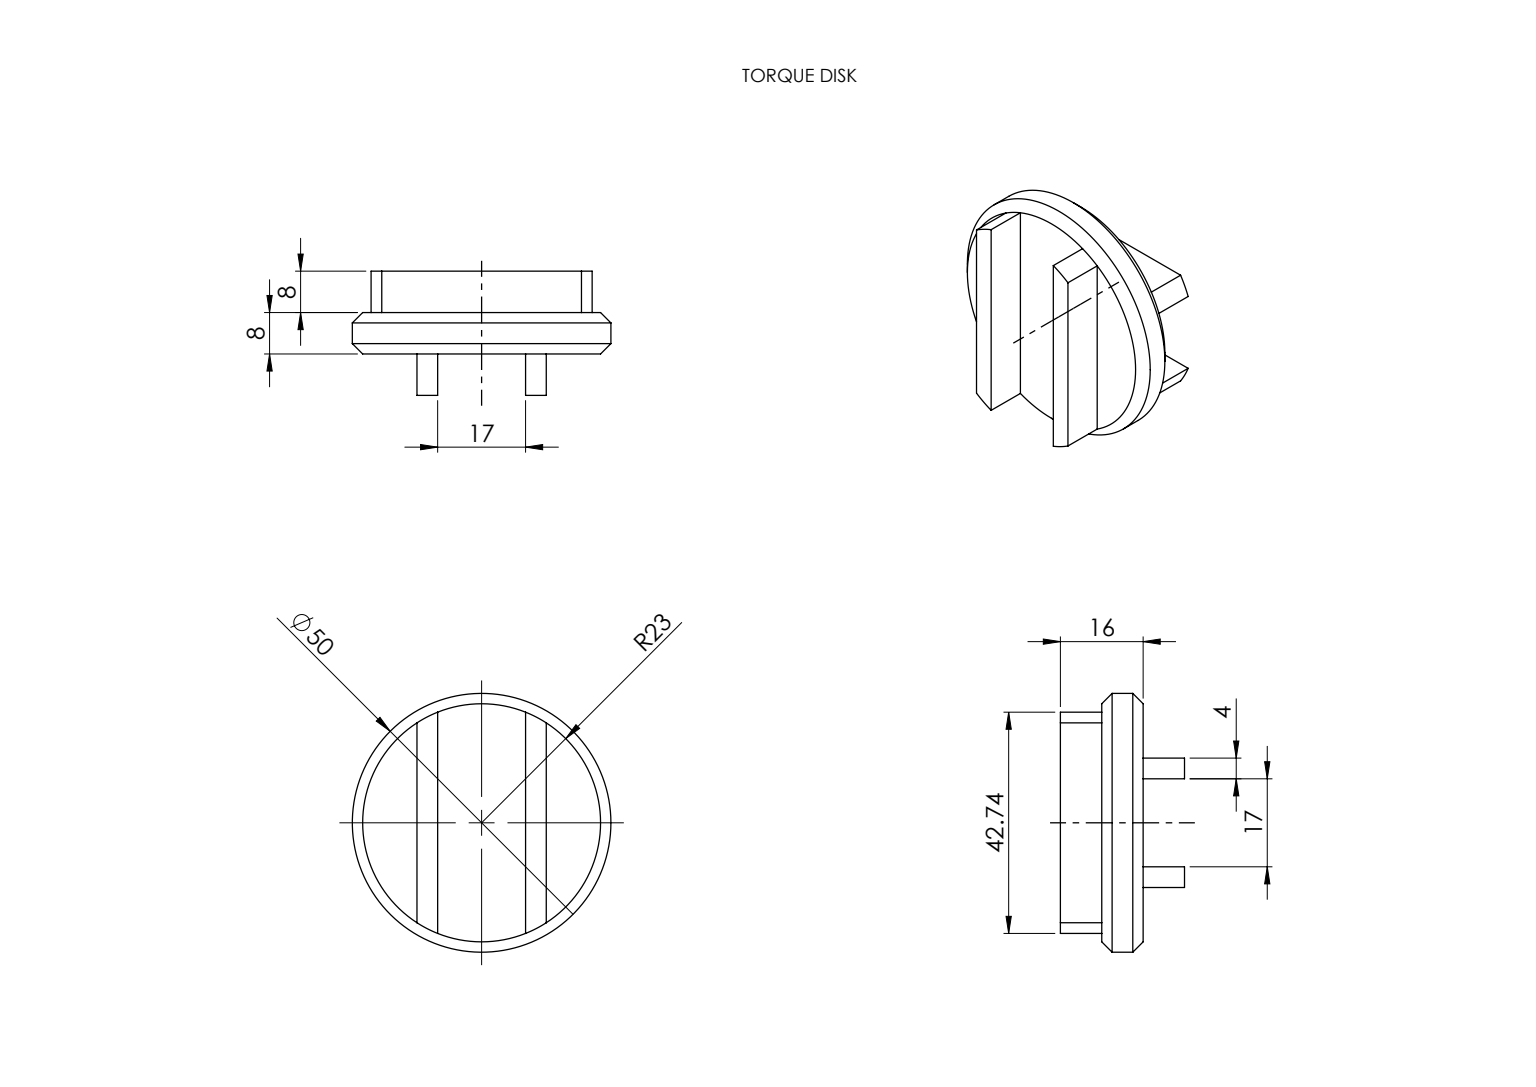
ISO-10303-21;
HEADER;
FILE_DESCRIPTION (('STEP AP214'),
    '1' );
FILE_NAME ('torque disk.step',
    '2026-10-08T14:09:18',
    ( '' ),
    ( '' ),
    'SwSTEP 2.0',
    'SolidWorks 2026',
    '' );
FILE_SCHEMA (( 'AUTOMOTIVE_DESIGN' ));
ENDSEC;

DATA;
#10=( NAMED_UNIT ( * ) PLANE_ANGLE_UNIT ( ) SI_UNIT ( $, .RADIAN. ) );
#11=EDGE_CURVE ( 'NONE', #1059, #406, #4156, .T. ) ;
#17=AXIS2_PLACEMENT_3D ( 'NONE', #2780, #4294, #3843 ) ;
#18=ADVANCED_FACE ( 'NONE', ( #4455 ), #1426, .T. ) ;
#30=ORIENTED_EDGE ( 'NONE', *, *, #808, .T. ) ;
#35=CIRCLE ( 'NONE', #4595, 22.99999999999998934 ) ;
#38=ADVANCED_BREP_SHAPE_REPRESENTATION ( '', ( #2058, #1918 ), #1039 ) ;
#53=EDGE_CURVE ( 'NONE', #754, #3692, #3957, .T. ) ;
#55=ORIENTED_EDGE ( 'NONE', *, *, #2270, .T. ) ;
#61=( NAMED_UNIT ( * ) PLANE_ANGLE_UNIT ( ) SI_UNIT ( $, .RADIAN. ) );
#62=CARTESIAN_POINT ( 'NONE',  ( 0.000000000000000000, 0.000000000000000000, 4.000000000000000000 ) ) ;
#68=EDGE_LOOP ( 'NONE', ( #4400, #3556, #1967, #1620 ) ) ;
#75=ORIENTED_EDGE ( 'NONE', *, *, #4606, .T. ) ;
#76=AXIS2_PLACEMENT_3D ( 'NONE', #1953, #1896, #4546 ) ;
#77=EDGE_LOOP ( 'NONE', ( #2842, #2826, #4730, #3841 ) ) ;
#78=EDGE_CURVE ( 'NONE', #3692, #754, #3167, .T. ) ;
#86=DIRECTION ( 'NONE',  ( 1.000000000000000000, 0.000000000000000000, -0.000000000000000000 ) ) ;
#93=LINE ( 'NONE', #2056, #2959 ) ;
#96=VECTOR ( 'NONE', #306, 1000.000000000000000 ) ;
#119=DIRECTION ( 'NONE',  ( 1.000000000000000000, 0.000000000000000000, 0.000000000000000000 ) ) ;
#123=DIRECTION ( 'NONE',  ( -0.000000000000000000, -0.000000000000000000, -1.000000000000000000 ) ) ;
#125=EDGE_LOOP ( 'NONE', ( #685, #558, #2484, #4035, #4209, #3718, #4513, #747 ) ) ;
#134=DIRECTION ( 'NONE',  ( 0.7071067811865487940, 0.000000000000000000, 0.7071067811865463515 ) ) ;
#152=ORIENTED_EDGE ( 'NONE', *, *, #1724, .T. ) ;
#167=CARTESIAN_POINT ( 'NONE',  ( -12.50000000000000178, 19.30673457630782863, 4.000000000000000000 ) ) ;
#169=AXIS2_PLACEMENT_3D ( 'NONE', #62, #3894, #4293 ) ;
#179=CARTESIAN_POINT ( 'NONE',  ( 23.00000000000000711, 2.939152317953648289E-15, 4.000000000000000000 ) ) ;
#186=DIRECTION ( 'NONE',  ( 1.000000000000000000, -1.106769389831504189E-16, 0.000000000000000000 ) ) ;
#192=ORIENTED_EDGE ( 'NONE', *, *, #1976, .T. ) ;
#200=DIRECTION ( 'NONE',  ( 1.000000000000000000, 0.000000000000000000, 0.000000000000000000 ) ) ;
#203=CARTESIAN_POINT ( 'NONE',  ( 2.853620410115562697E-14, 8.500000000000001776, -12.00000000000000000 ) ) ;
#205=CARTESIAN_POINT ( 'NONE',  ( 0.000000000000000000, 0.000000000000000000, -12.00000000000000000 ) ) ;
#212=VERTEX_POINT ( 'NONE', #756 ) ;
#215=DIRECTION ( 'NONE',  ( -0.000000000000000000, 0.000000000000000000, 1.000000000000000000 ) ) ;
#224=DIRECTION ( 'NONE',  ( -0.000000000000000000, -0.000000000000000000, 1.000000000000000000 ) ) ;
#234=EDGE_CURVE ( 'NONE', #1400, #1443, #448, .T. ) ;
#235=EDGE_LOOP ( 'NONE', ( #4089, #4144 ) ) ;
#246=ORIENTED_EDGE ( 'NONE', *, *, #3864, .T. ) ;
#257=AXIS2_PLACEMENT_3D ( 'NONE', #3512, #3491, #493 ) ;
#272=EDGE_CURVE ( 'NONE', #4859, #4459, #35, .T. ) ;
#283=ORIENTED_EDGE ( 'NONE', *, *, #1551, .T. ) ;
#287=ORIENTED_EDGE ( 'NONE', *, *, #3972, .T. ) ;
#291=DIRECTION ( 'NONE',  ( -1.106769389831504682E-16, -1.000000000000000000, 0.000000000000000000 ) ) ;
#293=FACE_OUTER_BOUND ( 'NONE', #4691, .T. ) ;
#301=CARTESIAN_POINT ( 'NONE',  ( 0.000000000000000000, 0.000000000000000000, 12.00000000000000000 ) ) ;
#302=CARTESIAN_POINT ( 'NONE',  ( 0.000000000000000000, 0.000000000000000000, -12.00000000000000000 ) ) ;
#306=DIRECTION ( 'NONE',  ( 1.000000000000000000, -3.578554360455197734E-15, 0.000000000000000000 ) ) ;
#308=ORIENTED_EDGE ( 'NONE', *, *, #4604, .F. ) ;
#320=PLANE ( 'NONE',  #4355 ) ;
#328=DIRECTION ( 'NONE',  ( -0.000000000000000000, -0.000000000000000000, 1.000000000000000000 ) ) ;
#333=DIRECTION ( 'NONE',  ( 0.000000000000000000, 0.000000000000000000, 1.000000000000000000 ) ) ;
#337=VECTOR ( 'NONE', #2303, 999.9999999999998863 ) ;
#352=ADVANCED_FACE ( 'NONE', ( #4835 ), #4072, .F. ) ;
#372=DIRECTION ( 'NONE',  ( 0.000000000000000000, 0.000000000000000000, 1.000000000000000000 ) ) ;
#374=VERTEX_POINT ( 'NONE', #1802 ) ;
#379=EDGE_CURVE ( 'NONE', #803, #3915, #997, .T. ) ;
#384=DIRECTION ( 'NONE',  ( 1.000000000000000000, -3.578554360455197734E-15, 0.000000000000000000 ) ) ;
#403=CYLINDRICAL_SURFACE ( 'NONE', #418, 23.00000000000000711 ) ;
#406=VERTEX_POINT ( 'NONE', #2208 ) ;
#412=CARTESIAN_POINT ( 'NONE',  ( 0.000000000000000000, 0.000000000000000000, -1.999999999999994893 ) ) ;
#417=FILL_AREA_STYLE ('',( #3127 ) ) ;
#418=AXIS2_PLACEMENT_3D ( 'NONE', #1930, #2739, #4659 ) ;
#421=ADVANCED_FACE ( 'NONE', ( #3011 ), #320, .F. ) ;
#422=DIRECTION ( 'NONE',  ( -0.000000000000000000, -0.000000000000000000, 1.000000000000000000 ) ) ;
#430=EDGE_CURVE ( 'NONE', #3154, #4346, #3398, .T. ) ;
#439=DIRECTION ( 'NONE',  ( -0.000000000000000000, -0.000000000000000000, 1.000000000000000000 ) ) ;
#440=DIRECTION ( 'NONE',  ( 0.000000000000000000, 0.000000000000000000, 1.000000000000000000 ) ) ;
#442=EDGE_LOOP ( 'NONE', ( #1911, #3869, #3953, #75 ) ) ;
#444=DIRECTION ( 'NONE',  ( -0.000000000000000000, -0.000000000000000000, -1.000000000000000000 ) ) ;
#445=CARTESIAN_POINT ( 'NONE',  ( 0.000000000000000000, 0.000000000000000000, -12.00000000000000000 ) ) ;
#448=CIRCLE ( 'NONE', #1077, 22.99999999999998934 ) ;
#450=EDGE_CURVE ( 'NONE', #1059, #4052, #4677, .T. ) ;
#451=VERTEX_POINT ( 'NONE', #717 ) ;
#453=CARTESIAN_POINT ( 'NONE',  ( 0.000000000000000000, 0.000000000000000000, 4.000000000000000000 ) ) ;
#454=DIRECTION ( 'NONE',  ( -0.000000000000000000, 0.000000000000000000, 1.000000000000000000 ) ) ;
#456=ORIENTED_EDGE ( 'NONE', *, *, #4832, .F. ) ;
#458=LINE ( 'NONE', #766, #3279 ) ;
#470=CARTESIAN_POINT ( 'NONE',  ( 12.50000000000000178, 19.30673457630782863, 12.00000000000000000 ) ) ;
#471=FACE_OUTER_BOUND ( 'NONE', #854, .T. ) ;
#490=LINE ( 'NONE', #2006, #2180 ) ;
#493=DIRECTION ( 'NONE',  ( 1.000000000000000000, 0.000000000000000000, -0.000000000000000000 ) ) ;
#499=ORIENTED_EDGE ( 'NONE', *, *, #2997, .T. ) ;
#501=CARTESIAN_POINT ( 'NONE',  ( -12.49999999999999822, -19.30673457630782863, 12.00000000000000000 ) ) ;
#505=AXIS2_PLACEMENT_3D ( 'NONE', #2463, #2918, #1335 ) ;
#514=CARTESIAN_POINT ( 'NONE',  ( 8.500000000000003553, 21.37171027316251681, 12.00000000000000000 ) ) ;
#533=ORIENTED_EDGE ( 'NONE', *, *, #715, .T. ) ;
#535=EDGE_CURVE ( 'NONE', #1202, #406, #2812, .T. ) ;
#542=ORIENTED_EDGE ( 'NONE', *, *, #78, .F. ) ;
#548=EDGE_CURVE ( 'NONE', #3988, #553, #2328, .T. ) ;
#550=FACE_OUTER_BOUND ( 'NONE', #3936, .T. ) ;
#553=VERTEX_POINT ( 'NONE', #4700 ) ;
#556=DIRECTION ( 'NONE',  ( 1.000000000000000000, 0.000000000000000000, 0.000000000000000000 ) ) ;
#558=ORIENTED_EDGE ( 'NONE', *, *, #1089, .T. ) ;
#562=ORIENTED_EDGE ( 'NONE', *, *, #3354, .F. ) ;
#568=CARTESIAN_POINT ( 'NONE',  ( 0.000000000000000000, 0.000000000000000000, -4.000000000000000000 ) ) ;
#578=VECTOR ( 'NONE', #4525, 1000.000000000000000 ) ;
#581=DIRECTION ( 'NONE',  ( 1.000000000000000000, -3.578554360455197734E-15, 0.000000000000000000 ) ) ;
#585=CIRCLE ( 'NONE', #1233, 22.99999999999998934 ) ;
#590=CARTESIAN_POINT ( 'NONE',  ( 2.853620410115562697E-14, 8.500000000000001776, -4.000000000000000000 ) ) ;
#614=DIRECTION ( 'NONE',  ( -1.000000000000000000, 0.000000000000000000, -0.000000000000000000 ) ) ;
#634=DIRECTION ( 'NONE',  ( 1.000000000000000000, 0.000000000000000000, 0.000000000000000000 ) ) ;
#635=ORIENTED_EDGE ( 'NONE', *, *, #379, .F. ) ;
#639=AXIS2_PLACEMENT_3D ( 'NONE', #2764, #2840, #2031 ) ;
#647=VECTOR ( 'NONE', #648, 1000.000000000000000 ) ;
#648=DIRECTION ( 'NONE',  ( -0.000000000000000000, -0.000000000000000000, 1.000000000000000000 ) ) ;
#650=CARTESIAN_POINT ( 'NONE',  ( 8.500000000000000000, -21.37171027316251681, 12.00000000000000000 ) ) ;
#652=VECTOR ( 'NONE', #2590, 1000.000000000000000 ) ;
#667=LINE ( 'NONE', #3029, #2342 ) ;
#677=DIRECTION ( 'NONE',  ( 0.000000000000000000, 0.000000000000000000, 1.000000000000000000 ) ) ;
#678=CARTESIAN_POINT ( 'NONE',  ( -12.50000000000000178, 19.30673457630782863, 12.00000000000000000 ) ) ;
#683=CARTESIAN_POINT ( 'NONE',  ( -3.041771206386918902E-14, -8.500000000000001776, -4.000000000000000000 ) ) ;
#685=ORIENTED_EDGE ( 'NONE', *, *, #4356, .F. ) ;
#691=DIRECTION ( 'NONE',  ( -1.000000000000000000, 0.000000000000000000, 0.000000000000000000 ) ) ;
#697=ORIENTED_EDGE ( 'NONE', *, *, #53, .T. ) ;
#712=( NAMED_UNIT ( * ) SI_UNIT ( $, .STERADIAN. ) SOLID_ANGLE_UNIT ( ) );
#715=EDGE_CURVE ( 'NONE', #2919, #4243, #4022, .T. ) ;
#717=CARTESIAN_POINT ( 'NONE',  ( -19.30673457630776824, 12.50000000000006750, -12.00000000000000000 ) ) ;
#725=FACE_OUTER_BOUND ( 'NONE', #235, .T. ) ;
#728=AXIS2_PLACEMENT_3D ( 'NONE', #4369, #3714, #4113 ) ;
#743=VECTOR ( 'NONE', #4151, 1000.000000000000000 ) ;
#745=AXIS2_PLACEMENT_3D ( 'NONE', #2471, #215, #119 ) ;
#747=ORIENTED_EDGE ( 'NONE', *, *, #1982, .F. ) ;
#750=CARTESIAN_POINT ( 'NONE',  ( 0.000000000000000000, 0.000000000000000000, -12.00000000000000000 ) ) ;
#753=CARTESIAN_POINT ( 'NONE',  ( -8.500000000000001776, -9.407539813567788568E-16, 12.00000000000000000 ) ) ;
#754=VERTEX_POINT ( 'NONE', #3235 ) ;
#756=CARTESIAN_POINT ( 'NONE',  ( 21.37171027316252747, 8.499999999999930722, -12.00000000000000000 ) ) ;
#760=ORIENTED_EDGE ( 'NONE', *, *, #4860, .T. ) ;
#766=CARTESIAN_POINT ( 'NONE',  ( 2.853620410115562697E-14, 8.500000000000001776, -12.00000000000000000 ) ) ;
#767=DIRECTION ( 'NONE',  ( 1.000000000000000000, 0.000000000000000000, -0.000000000000000000 ) ) ;
#785=ORIENTED_EDGE ( 'NONE', *, *, #1577, .T. ) ;
#793=AXIS2_PLACEMENT_3D ( 'NONE', #568, #872, #200 ) ;
#795=ORIENTED_EDGE ( 'NONE', *, *, #4142, .T. ) ;
#802=EDGE_CURVE ( 'NONE', #1443, #1649, #1414, .T. ) ;
#803=VERTEX_POINT ( 'NONE', #2455 ) ;
#808=EDGE_CURVE ( 'NONE', #4311, #4747, #3622, .T. ) ;
#820=EDGE_CURVE ( 'NONE', #4459, #803, #4874, .T. ) ;
#823=( GEOMETRIC_REPRESENTATION_CONTEXT ( 3 ) GLOBAL_UNCERTAINTY_ASSIGNED_CONTEXT ( ( #1800 ) ) GLOBAL_UNIT_ASSIGNED_CONTEXT ( ( #4904, #2244, #712 ) ) REPRESENTATION_CONTEXT ( 'NONE', 'WORKASPACE' ) );
#836=VECTOR ( 'NONE', #2616, 1000.000000000000000 ) ;
#845=CARTESIAN_POINT ( 'NONE',  ( 0.000000000000000000, 0.000000000000000000, 4.000000000000000000 ) ) ;
#846=CARTESIAN_POINT ( 'NONE',  ( 25.00000000000000000, 3.061616997868383043E-15, 2.000000000000001776 ) ) ;
#854=EDGE_LOOP ( 'NONE', ( #2425, #1849, #2892, #2036 ) ) ;
#858=ORIENTED_EDGE ( 'NONE', *, *, #1121, .F. ) ;
#859=ORIENTED_EDGE ( 'NONE', *, *, #3629, .T. ) ;
#861=DIRECTION ( 'NONE',  ( 1.000000000000000000, 0.000000000000000000, 0.000000000000000000 ) ) ;
#871=ORIENTED_EDGE ( 'NONE', *, *, #3110, .F. ) ;
#872=DIRECTION ( 'NONE',  ( -0.000000000000000000, -0.000000000000000000, -1.000000000000000000 ) ) ;
#886=DIRECTION ( 'NONE',  ( -1.106769389831504682E-16, 1.000000000000000000, 0.000000000000000000 ) ) ;
#889=ORIENTED_EDGE ( 'NONE', *, *, #3864, .F. ) ;
#906=AXIS2_PLACEMENT_3D ( 'NONE', #1992, #422, #1970 ) ;
#907=EDGE_CURVE ( 'NONE', #553, #1430, #4192, .T. ) ;
#913=EDGE_CURVE ( 'NONE', #4443, #3659, #2973, .T. ) ;
#914=ADVANCED_FACE ( 'NONE', ( #4098 ), #1509, .T. ) ;
#917=FACE_OUTER_BOUND ( 'NONE', #4676, .T. ) ;
#920=ORIENTED_EDGE ( 'NONE', *, *, #3837, .F. ) ;
#923=FACE_OUTER_BOUND ( 'NONE', #3338, .T. ) ;
#933=EDGE_LOOP ( 'NONE', ( #1425, #3642, #1924, #2330 ) ) ;
#936=CARTESIAN_POINT ( 'NONE',  ( 12.50000000000000178, 19.30673457630782863, 12.00000000000000000 ) ) ;
#944=CARTESIAN_POINT ( 'NONE',  ( 0.000000000000000000, 0.000000000000000000, -1.999999999999994893 ) ) ;
#950=PRODUCT_CONTEXT ( 'NONE', #1025, 'mechanical' ) ;
#954=ADVANCED_FACE ( 'NONE', ( #3053 ), #4556, .T. ) ;
#955=DIRECTION ( 'NONE',  ( -1.000000000000000000, 0.000000000000000000, 0.000000000000000000 ) ) ;
#960=ORIENTED_EDGE ( 'NONE', *, *, #1121, .T. ) ;
#982=PLANE ( 'NONE',  #1299 ) ;
#983=AXIS2_PLACEMENT_3D ( 'NONE', #1773, #1399, #2552 ) ;
#993=DIRECTION ( 'NONE',  ( 0.000000000000000000, 0.000000000000000000, -1.000000000000000000 ) ) ;
#995=ORIENTED_EDGE ( 'NONE', *, *, #430, .T. ) ;
#997=CIRCLE ( 'NONE', #1245, 22.99999999999998934 ) ;
#1003=SURFACE_SIDE_STYLE ('',( #1916 ) ) ;
#1005=ORIENTED_EDGE ( 'NONE', *, *, #430, .F. ) ;
#1012=LINE ( 'NONE', #2522, #2333 ) ;
#1013=DIRECTION ( 'NONE',  ( -0.000000000000000000, -0.000000000000000000, -1.000000000000000000 ) ) ;
#1019=ADVANCED_FACE ( 'NONE', ( #1641 ), #3083, .T. ) ;
#1025=APPLICATION_CONTEXT ( 'automotive_design' ) ;
#1039=( GEOMETRIC_REPRESENTATION_CONTEXT ( 3 ) GLOBAL_UNCERTAINTY_ASSIGNED_CONTEXT ( ( #2653 ) ) GLOBAL_UNIT_ASSIGNED_CONTEXT ( ( #1392, #61, #3082 ) ) REPRESENTATION_CONTEXT ( 'NONE', 'WORKASPACE' ) );
#1040=DIRECTION ( 'NONE',  ( -0.000000000000000000, -0.000000000000000000, 1.000000000000000000 ) ) ;
#1047=DIRECTION ( 'NONE',  ( 1.000000000000000000, 0.000000000000000000, 0.000000000000000000 ) ) ;
#1057=CIRCLE ( 'NONE', #2909, 23.00000000000000711 ) ;
#1059=VERTEX_POINT ( 'NONE', #501 ) ;
#1062=CIRCLE ( 'NONE', #3459, 23.00000000000000711 ) ;
#1066=DIRECTION ( 'NONE',  ( 1.000000000000000000, -3.357200482488897685E-15, 0.000000000000000000 ) ) ;
#1070=CARTESIAN_POINT ( 'NONE',  ( 0.000000000000000000, 0.000000000000000000, -12.00000000000000000 ) ) ;
#1074=DIRECTION ( 'NONE',  ( 1.000000000000000000, 0.000000000000000000, 0.000000000000000000 ) ) ;
#1076=DIRECTION ( 'NONE',  ( 0.000000000000000000, 0.000000000000000000, -1.000000000000000000 ) ) ;
#1077=AXIS2_PLACEMENT_3D ( 'NONE', #4425, #2866, #3670 ) ;
#1088=CARTESIAN_POINT ( 'NONE',  ( -19.30673457630785350, -12.49999999999993250, -4.000000000000000000 ) ) ;
#1089=EDGE_CURVE ( 'NONE', #3611, #3692, #4672, .T. ) ;
#1095=EDGE_CURVE ( 'NONE', #1430, #3154, #1291, .T. ) ;
#1100=CARTESIAN_POINT ( 'NONE',  ( 19.30673457630784995, 12.49999999999993783, -12.00000000000000000 ) ) ;
#1104=FACE_OUTER_BOUND ( 'NONE', #1169, .T. ) ;
#1105=ORIENTED_EDGE ( 'NONE', *, *, #450, .T. ) ;
#1110=LINE ( 'NONE', #4845, #1369 ) ;
#1111=DIRECTION ( 'NONE',  ( -0.000000000000000000, -0.000000000000000000, -1.000000000000000000 ) ) ;
#1112=CARTESIAN_POINT ( 'NONE',  ( -19.30673457630785350, -12.49999999999993250, -12.00000000000000000 ) ) ;
#1115=DIRECTION ( 'NONE',  ( 1.000000000000000000, 0.000000000000000000, 0.000000000000000000 ) ) ;
#1121=EDGE_CURVE ( 'NONE', #4243, #3154, #2398, .T. ) ;
#1123=DIRECTION ( 'NONE',  ( -0.000000000000000000, 0.000000000000000000, 1.000000000000000000 ) ) ;
#1130=DIRECTION ( 'NONE',  ( 1.000000000000000000, 0.000000000000000000, 0.000000000000000000 ) ) ;
#1131=CARTESIAN_POINT ( 'NONE',  ( 0.000000000000000000, 0.000000000000000000, 4.000000000000000000 ) ) ;
#1134=CIRCLE ( 'NONE', #2576, 23.00000000000000711 ) ;
#1138=CARTESIAN_POINT ( 'NONE',  ( -8.500000000000000000, -21.37171027316251681, 12.00000000000000000 ) ) ;
#1146=CARTESIAN_POINT ( 'NONE',  ( 0.000000000000000000, 0.000000000000000000, 0.000000000000000000 ) ) ;
#1156=ORIENTED_EDGE ( 'NONE', *, *, #3546, .T. ) ;
#1157=AXIS2_PLACEMENT_3D ( 'NONE', #2564, #333, #4084 ) ;
#1167=DIRECTION ( 'NONE',  ( -1.000000000000000000, 0.000000000000000000, -0.000000000000000000 ) ) ;
#1169=EDGE_LOOP ( 'NONE', ( #2876, #3862, #4101, #2317 ) ) ;
#1175=PLANE ( 'NONE',  #3916 ) ;
#1180=ORIENTED_EDGE ( 'NONE', *, *, #2385, .F. ) ;
#1184=CARTESIAN_POINT ( 'NONE',  ( -23.00000000000000711, 0.000000000000000000, 4.000000000000000000 ) ) ;
#1199=FACE_OUTER_BOUND ( 'NONE', #77, .T. ) ;
#1201=AXIS2_PLACEMENT_3D ( 'NONE', #2326, #3108, #3403 ) ;
#1202=VERTEX_POINT ( 'NONE', #3638 ) ;
#1205=AXIS2_PLACEMENT_3D ( 'NONE', #2976, #4465, #4097 ) ;
#1212=VECTOR ( 'NONE', #4165, 1000.000000000000000 ) ;
#1233=AXIS2_PLACEMENT_3D ( 'NONE', #4436, #1013, #634 ) ;
#1236=DIRECTION ( 'NONE',  ( -1.000000000000000000, 0.000000000000000000, 0.000000000000000000 ) ) ;
#1238=EDGE_LOOP ( 'NONE', ( #152, #2360, #308, #499 ) ) ;
#1245=AXIS2_PLACEMENT_3D ( 'NONE', #3331, #4858, #1047 ) ;
#1250=DIRECTION ( 'NONE',  ( 0.000000000000000000, 0.000000000000000000, -1.000000000000000000 ) ) ;
#1255=CARTESIAN_POINT ( 'NONE',  ( 0.000000000000000000, 0.000000000000000000, 4.000000000000000000 ) ) ;
#1260=DIRECTION ( 'NONE',  ( -0.000000000000000000, -0.000000000000000000, -1.000000000000000000 ) ) ;
#1262=VERTEX_POINT ( 'NONE', #2170 ) ;
#1275=DIRECTION ( 'NONE',  ( 0.000000000000000000, 0.000000000000000000, 1.000000000000000000 ) ) ;
#1282=DIRECTION ( 'NONE',  ( 1.000000000000000000, 0.000000000000000000, 0.000000000000000000 ) ) ;
#1291=CIRCLE ( 'NONE', #169, 23.00000000000000711 ) ;
#1299=AXIS2_PLACEMENT_3D ( 'NONE', #3607, #186, #4006 ) ;
#1301=CARTESIAN_POINT ( 'NONE',  ( 0.000000000000000000, 0.000000000000000000, 12.00000000000000000 ) ) ;
#1313=VERTEX_POINT ( 'NONE', #1340 ) ;
#1325=DIRECTION ( 'NONE',  ( -0.7071067811865487940, 8.659560562354948882E-17, 0.7071067811865463515 ) ) ;
#1335=DIRECTION ( 'NONE',  ( 1.000000000000000000, -3.357200482488897685E-15, 0.000000000000000000 ) ) ;
#1338=ADVANCED_FACE ( 'NONE', ( #2859 ), #3251, .T. ) ;
#1340=CARTESIAN_POINT ( 'NONE',  ( -21.37171027316253102, -8.499999999999925393, -12.00000000000000000 ) ) ;
#1344=DIRECTION ( 'NONE',  ( -1.000000000000000000, 0.000000000000000000, 0.000000000000000000 ) ) ;
#1348=ORIENTED_EDGE ( 'NONE', *, *, #78, .T. ) ;
#1359=DIRECTION ( 'NONE',  ( 1.000000000000000000, 0.000000000000000000, 0.000000000000000000 ) ) ;
#1369=VECTOR ( 'NONE', #1501, 1000.000000000000000 ) ;
#1373=AXIS2_PLACEMENT_3D ( 'NONE', #4363, #2088, #955 ) ;
#1385=EDGE_CURVE ( 'NONE', #451, #3363, #1110, .T. ) ;
#1391=ORIENTED_EDGE ( 'NONE', *, *, #3477, .T. ) ;
#1392=( LENGTH_UNIT ( ) NAMED_UNIT ( * ) SI_UNIT ( .MILLI., .METRE. ) );
#1398=DIRECTION ( 'NONE',  ( 3.357200482488897290E-15, 1.000000000000000000, 0.000000000000000000 ) ) ;
#1399=DIRECTION ( 'NONE',  ( -0.000000000000000000, -0.000000000000000000, 1.000000000000000000 ) ) ;
#1400=VERTEX_POINT ( 'NONE', #4134 ) ;
#1402=CARTESIAN_POINT ( 'NONE',  ( -3.041771206386918902E-14, -8.500000000000001776, -12.00000000000000000 ) ) ;
#1403=CARTESIAN_POINT ( 'NONE',  ( 0.000000000000000000, 0.000000000000000000, 4.000000000000000000 ) ) ;
#1409=CARTESIAN_POINT ( 'NONE',  ( -4.473192950568998942E-14, -12.50000000000000178, -4.000000000000000000 ) ) ;
#1414=LINE ( 'NONE', #4353, #2649 ) ;
#1416=ORIENTED_EDGE ( 'NONE', *, *, #1982, .T. ) ;
#1419=DIRECTION ( 'NONE',  ( -1.000000000000000000, 0.000000000000000000, 0.000000000000000000 ) ) ;
#1425=ORIENTED_EDGE ( 'NONE', *, *, #3837, .T. ) ;
#1426=PLANE ( 'NONE',  #1157 ) ;
#1429=LINE ( 'NONE', #2972, #2189 ) ;
#1430=VERTEX_POINT ( 'NONE', #2193 ) ;
#1443=VERTEX_POINT ( 'NONE', #3319 ) ;
#1444=VECTOR ( 'NONE', #439, 1000.000000000000000 ) ;
#1448=PLANE ( 'NONE',  #4897 ) ;
#1450=DIRECTION ( 'NONE',  ( 1.000000000000000000, 0.000000000000000000, 0.000000000000000000 ) ) ;
#1453=AXIS2_PLACEMENT_3D ( 'NONE', #4587, #440, #2284 ) ;
#1454=COLOUR_RGB ( '', 0.40784314, 0.44705882, 0.49803922) ;
#1464=FACE_OUTER_BOUND ( 'NONE', #442, .T. ) ;
#1465=DIRECTION ( 'NONE',  ( -0.000000000000000000, -0.000000000000000000, -1.000000000000000000 ) ) ;
#1482=CARTESIAN_POINT ( 'NONE',  ( 21.37171027316246708, -8.500000000000078160, -12.00000000000000000 ) ) ;
#1488=CARTESIAN_POINT ( 'NONE',  ( 19.30673457630776468, -12.50000000000007105, -12.00000000000000000 ) ) ;
#1501=DIRECTION ( 'NONE',  ( 1.000000000000000000, -3.357200482488897685E-15, 0.000000000000000000 ) ) ;
#1503=DIRECTION ( 'NONE',  ( -0.000000000000000000, -0.000000000000000000, 1.000000000000000000 ) ) ;
#1505=CIRCLE ( 'NONE', #1201, 22.99999999999998934 ) ;
#1507=SURFACE_STYLE_FILL_AREA ( #417 ) ;
#1509=CYLINDRICAL_SURFACE ( 'NONE', #3846, 25.00000000000000000 ) ;
#1523=CYLINDRICAL_SURFACE ( 'NONE', #4895, 23.00000000000000711 ) ;
#1530=CARTESIAN_POINT ( 'NONE',  ( 0.000000000000000000, 0.000000000000000000, 4.000000000000000000 ) ) ;
#1533=VECTOR ( 'NONE', #1659, 1000.000000000000000 ) ;
#1537=AXIS2_PLACEMENT_3D ( 'NONE', #750, #328, #1130 ) ;
#1538=STYLED_ITEM ( 'NONE', ( #3422 ), #2058 ) ;
#1542=VECTOR ( 'NONE', #291, 1000.000000000000000 ) ;
#1548=DIRECTION ( 'NONE',  ( 0.000000000000000000, 0.000000000000000000, 1.000000000000000000 ) ) ;
#1551=EDGE_CURVE ( 'NONE', #4747, #1202, #3934, .T. ) ;
#1556=CARTESIAN_POINT ( 'NONE',  ( 0.000000000000000000, 0.000000000000000000, 12.00000000000000000 ) ) ;
#1563=ORIENTED_EDGE ( 'NONE', *, *, #3872, .T. ) ;
#1571=ADVANCED_FACE ( 'NONE', ( #2795 ), #1606, .T. ) ;
#1574=EDGE_CURVE ( 'NONE', #3659, #2525, #1768, .T. ) ;
#1575=DIRECTION ( 'NONE',  ( -0.000000000000000000, -0.000000000000000000, 1.000000000000000000 ) ) ;
#1577=EDGE_CURVE ( 'NONE', #2525, #803, #3220, .T. ) ;
#1586=ORIENTED_EDGE ( 'NONE', *, *, #2131, .T. ) ;
#1587=PRESENTATION_STYLE_ASSIGNMENT (( #2242 ) ) ;
#1589=DIRECTION ( 'NONE',  ( 1.000000000000000000, 0.000000000000000000, 0.000000000000000000 ) ) ;
#1591=ORIENTED_EDGE ( 'NONE', *, *, #3546, .F. ) ;
#1594=VERTEX_POINT ( 'NONE', #470 ) ;
#1596=ADVANCED_FACE ( 'NONE', ( #3076 ), #1964, .T. ) ;
#1606=CYLINDRICAL_SURFACE ( 'NONE', #3849, 25.00000000000000000 ) ;
#1613=ORIENTED_EDGE ( 'NONE', *, *, #913, .T. ) ;
#1616=DIRECTION ( 'NONE',  ( 0.7071067811865469066, 8.659560562354926695E-17, -0.7071067811865482389 ) ) ;
#1620=ORIENTED_EDGE ( 'NONE', *, *, #1095, .T. ) ;
#1623=DIRECTION ( 'NONE',  ( -0.000000000000000000, -0.000000000000000000, 1.000000000000000000 ) ) ;
#1625=CIRCLE ( 'NONE', #2753, 22.99999999999998934 ) ;
#1639=EDGE_LOOP ( 'NONE', ( #995, #871, #2214, #960 ) ) ;
#1641=FACE_OUTER_BOUND ( 'NONE', #68, .T. ) ;
#1644=SHAPE_REPRESENTATION ( 'torque disk', ( #1918 ), #1039 ) ;
#1648=DIRECTION ( 'NONE',  ( 1.000000000000000000, 0.000000000000000000, 0.000000000000000000 ) ) ;
#1649=VERTEX_POINT ( 'NONE', #3263 ) ;
#1657=PLANE ( 'NONE',  #3771 ) ;
#1659=DIRECTION ( 'NONE',  ( -0.000000000000000000, -0.000000000000000000, 1.000000000000000000 ) ) ;
#1668=PRODUCT ( 'torque disk', 'torque disk', '', ( #950 ) ) ;
#1677=CARTESIAN_POINT ( 'NONE',  ( 0.000000000000000000, 0.000000000000000000, 4.000000000000000000 ) ) ;
#1679=ORIENTED_EDGE ( 'NONE', *, *, #3629, .F. ) ;
#1702=EDGE_LOOP ( 'NONE', ( #2064, #1591, #562, #795 ) ) ;
#1708=ORIENTED_EDGE ( 'NONE', *, *, #3725, .F. ) ;
#1711=CARTESIAN_POINT ( 'NONE',  ( -21.37171027316247063, 8.500000000000072831, -12.00000000000000000 ) ) ;
#1723=APPLICATION_CONTEXT ( 'automotive_design' ) ;
#1724=EDGE_CURVE ( 'NONE', #3915, #1400, #3539, .T. ) ;
#1726=ADVANCED_FACE ( 'NONE', ( #4005 ), #1657, .F. ) ;
#1736=EDGE_LOOP ( 'NONE', ( #2085, #3107, #889, #2894, #3323, #3821, #3521, #1708 ) ) ;
#1742=SHAPE_DEFINITION_REPRESENTATION ( #3097, #1644 ) ;
#1748=FACE_OUTER_BOUND ( 'NONE', #3830, .T. ) ;
#1751=ORIENTED_EDGE ( 'NONE', *, *, #1883, .T. ) ;
#1753=ORIENTED_EDGE ( 'NONE', *, *, #4263, .T. ) ;
#1759=VECTOR ( 'NONE', #1837, 1000.000000000000000 ) ;
#1768=CIRCLE ( 'NONE', #4649, 22.99999999999998934 ) ;
#1773=CARTESIAN_POINT ( 'NONE',  ( 0.000000000000000000, 0.000000000000000000, -1.999999999999994893 ) ) ;
#1780=CIRCLE ( 'NONE', #3547, 23.00000000000000711 ) ;
#1782=EDGE_LOOP ( 'NONE', ( #55, #4725, #4647, #30 ) ) ;
#1800=UNCERTAINTY_MEASURE_WITH_UNIT (LENGTH_MEASURE( 1.000000000000000082E-05 ), #4904, 'distance_accuracy_value', 'NONE');
#1802=CARTESIAN_POINT ( 'NONE',  ( -19.30673457630776824, 12.50000000000006750, -4.000000000000000000 ) ) ;
#1804=EDGE_LOOP ( 'NONE', ( #1416, #4432, #4933, #2635 ) ) ;
#1818=DIRECTION ( 'NONE',  ( 1.000000000000000000, 5.329070518200750605E-15, 0.000000000000000000 ) ) ;
#1821=( GEOMETRIC_REPRESENTATION_CONTEXT ( 3 ) GLOBAL_UNCERTAINTY_ASSIGNED_CONTEXT ( ( #4602 ) ) GLOBAL_UNIT_ASSIGNED_CONTEXT ( ( #3420, #10, #3813 ) ) REPRESENTATION_CONTEXT ( 'NONE', 'WORKASPACE' ) );
#1827=LINE ( 'NONE', #1402, #96 ) ;
#1834=CIRCLE ( 'NONE', #2324, 22.99999999999998934 ) ;
#1837=DIRECTION ( 'NONE',  ( -0.000000000000000000, -0.000000000000000000, 1.000000000000000000 ) ) ;
#1847=VECTOR ( 'NONE', #134, 1000.000000000000000 ) ;
#1849=ORIENTED_EDGE ( 'NONE', *, *, #3355, .T. ) ;
#1856=PLANE ( 'NONE',  #1453 ) ;
#1858=CIRCLE ( 'NONE', #17, 23.00000000000000711 ) ;
#1862=LINE ( 'NONE', #1482, #1943 ) ;
#1863=LINE ( 'NONE', #2567, #1542 ) ;
#1868=SURFACE_STYLE_USAGE ( .BOTH. , #1003 ) ;
#1869=ORIENTED_EDGE ( 'NONE', *, *, #234, .T. ) ;
#1870=AXIS2_PLACEMENT_3D ( 'NONE', #2169, #2968, #4529 ) ;
#1871=ADVANCED_FACE ( 'NONE', ( #4107 ), #1448, .F. ) ;
#1881=PLANE ( 'NONE',  #4575 ) ;
#1882=ORIENTED_EDGE ( 'NONE', *, *, #3560, .F. ) ;
#1883=EDGE_CURVE ( 'NONE', #3363, #2945, #2587, .T. ) ;
#1896=DIRECTION ( 'NONE',  ( 1.000000000000000000, -1.106769389831504682E-16, 0.000000000000000000 ) ) ;
#1898=ORIENTED_EDGE ( 'NONE', *, *, #2997, .F. ) ;
#1911=ORIENTED_EDGE ( 'NONE', *, *, #3354, .T. ) ;
#1916=SURFACE_STYLE_FILL_AREA ( #2295 ) ;
#1918=AXIS2_PLACEMENT_3D ( 'NONE', #1146, #2700, #1115 ) ;
#1922=AXIS2_PLACEMENT_3D ( 'NONE', #1255, #1275, #1648 ) ;
#1924=ORIENTED_EDGE ( 'NONE', *, *, #4606, .F. ) ;
#1930=CARTESIAN_POINT ( 'NONE',  ( 0.000000000000000000, 0.000000000000000000, 12.00000000000000000 ) ) ;
#1943=VECTOR ( 'NONE', #4114, 1000.000000000000000 ) ;
#1953=CARTESIAN_POINT ( 'NONE',  ( 12.50000000000000000, -1.383461737289380927E-15, 12.00000000000000000 ) ) ;
#1956=ORIENTED_EDGE ( 'NONE', *, *, #4263, .F. ) ;
#1964=PLANE ( 'NONE',  #257 ) ;
#1967=ORIENTED_EDGE ( 'NONE', *, *, #907, .T. ) ;
#1970=DIRECTION ( 'NONE',  ( 1.000000000000000000, 0.000000000000000000, 0.000000000000000000 ) ) ;
#1973=CARTESIAN_POINT ( 'NONE',  ( 0.000000000000000000, 0.000000000000000000, -4.000000000000000000 ) ) ;
#1975=ORIENTED_EDGE ( 'NONE', *, *, #808, .F. ) ;
#1976=EDGE_CURVE ( 'NONE', #2919, #3988, #3649, .T. ) ;
#1982=EDGE_CURVE ( 'NONE', #3321, #3988, #2661, .T. ) ;
#1984=ORIENTED_EDGE ( 'NONE', *, *, #1574, .F. ) ;
#1985=DIRECTION ( 'NONE',  ( 1.000000000000000000, 0.000000000000000000, 0.000000000000000000 ) ) ;
#1992=CARTESIAN_POINT ( 'NONE',  ( 0.000000000000000000, 0.000000000000000000, -12.00000000000000000 ) ) ;
#1998=ORIENTED_EDGE ( 'NONE', *, *, #820, .F. ) ;
#2006=CARTESIAN_POINT ( 'NONE',  ( 12.49999999999999822, -19.30673457630782863, 12.00000000000000000 ) ) ;
#2031=DIRECTION ( 'NONE',  ( 1.000000000000000000, 0.000000000000000000, 0.000000000000000000 ) ) ;
#2036=ORIENTED_EDGE ( 'NONE', *, *, #2816, .T. ) ;
#2038=DIRECTION ( 'NONE',  ( 1.000000000000000000, 0.000000000000000000, 0.000000000000000000 ) ) ;
#2039=LINE ( 'NONE', #3507, #4744 ) ;
#2045=LINE ( 'NONE', #3100, #1847 ) ;
#2051=CARTESIAN_POINT ( 'NONE',  ( 8.500000000000000000, -21.37171027316251681, 12.00000000000000000 ) ) ;
#2056=CARTESIAN_POINT ( 'NONE',  ( -21.37171027316253102, -8.499999999999925393, -12.00000000000000000 ) ) ;
#2058=MANIFOLD_SOLID_BREP ( 'Boss-Extrude3', #2915 ) ;
#2064=ORIENTED_EDGE ( 'NONE', *, *, #3725, .T. ) ;
#2068=FACE_OUTER_BOUND ( 'NONE', #1782, .T. ) ;
#2076=CYLINDRICAL_SURFACE ( 'NONE', #3040, 23.00000000000000711 ) ;
#2085=ORIENTED_EDGE ( 'NONE', *, *, #4797, .F. ) ;
#2088=DIRECTION ( 'NONE',  ( 0.000000000000000000, 0.000000000000000000, -1.000000000000000000 ) ) ;
#2099=DIRECTION ( 'NONE',  ( 1.000000000000000000, 0.000000000000000000, 0.000000000000000000 ) ) ;
#2101=ORIENTED_EDGE ( 'NONE', *, *, #2261, .F. ) ;
#2111=ADVANCED_FACE ( 'NONE', ( #3200 ), #3129, .T. ) ;
#2112=ADVANCED_FACE ( 'NONE', ( #3570 ), #3380, .T. ) ;
#2117=ORIENTED_EDGE ( 'NONE', *, *, #535, .F. ) ;
#2131=EDGE_CURVE ( 'NONE', #1594, #2919, #1858, .T. ) ;
#2144=ORIENTED_EDGE ( 'NONE', *, *, #234, .F. ) ;
#2149=ORIENTED_EDGE ( 'NONE', *, *, #1089, .F. ) ;
#2154=EDGE_LOOP ( 'NONE', ( #920, #1613, #2229, #4251, #1869, #4927 ) ) ;
#2169=CARTESIAN_POINT ( 'NONE',  ( 0.000000000000000000, 0.000000000000000000, 2.000000000000001776 ) ) ;
#2170=CARTESIAN_POINT ( 'NONE',  ( -21.37171027316247063, 8.500000000000072831, -4.000000000000000000 ) ) ;
#2174=CARTESIAN_POINT ( 'NONE',  ( 0.000000000000000000, 0.000000000000000000, -1.999999999999994893 ) ) ;
#2180=VECTOR ( 'NONE', #1260, 1000.000000000000000 ) ;
#2188=CARTESIAN_POINT ( 'NONE',  ( 8.500000000000003553, 21.37171027316251681, 12.00000000000000000 ) ) ;
#2189=VECTOR ( 'NONE', #1066, 1000.000000000000000 ) ;
#2192=AXIS2_PLACEMENT_3D ( 'NONE', #412, #1503, #4560 ) ;
#2193=CARTESIAN_POINT ( 'NONE',  ( -8.500000000000000000, -21.37171027316251681, 4.000000000000000000 ) ) ;
#2197=ADVANCED_FACE ( 'NONE', ( #923 ), #2724, .T. ) ;
#2208=CARTESIAN_POINT ( 'NONE',  ( -12.49999999999999822, -19.30673457630782863, 4.000000000000000000 ) ) ;
#2214=ORIENTED_EDGE ( 'NONE', *, *, #4204, .F. ) ;
#2216=EDGE_CURVE ( 'NONE', #212, #4443, #2878, .T. ) ;
#2223=CARTESIAN_POINT ( 'NONE',  ( 0.000000000000000000, 0.000000000000000000, -4.000000000000000000 ) ) ;
#2229=ORIENTED_EDGE ( 'NONE', *, *, #1574, .T. ) ;
#2242=SURFACE_STYLE_USAGE ( .BOTH. , #4191 ) ;
#2243=DIRECTION ( 'NONE',  ( -0.000000000000000000, -0.000000000000000000, -1.000000000000000000 ) ) ;
#2244=( NAMED_UNIT ( * ) PLANE_ANGLE_UNIT ( ) SI_UNIT ( $, .RADIAN. ) );
#2247=AXIS2_PLACEMENT_3D ( 'NONE', #4120, #4953, #691 ) ;
#2261=EDGE_CURVE ( 'NONE', #4758, #4052, #1012, .T. ) ;
#2263=ORIENTED_EDGE ( 'NONE', *, *, #3355, .F. ) ;
#2270=EDGE_CURVE ( 'NONE', #4747, #406, #2923, .T. ) ;
#2274=AXIS2_PLACEMENT_3D ( 'NONE', #3074, #3168, #2310 ) ;
#2276=EDGE_CURVE ( 'NONE', #3321, #4346, #3639, .T. ) ;
#2282=FACE_OUTER_BOUND ( 'NONE', #1238, .T. ) ;
#2283=CARTESIAN_POINT ( 'NONE',  ( 19.30673457630784995, 12.49999999999993783, -4.000000000000000000 ) ) ;
#2284=DIRECTION ( 'NONE',  ( 1.000000000000000000, 0.000000000000000000, -0.000000000000000000 ) ) ;
#2285=ORIENTED_EDGE ( 'NONE', *, *, #2412, .F. ) ;
#2292=ORIENTED_EDGE ( 'NONE', *, *, #3572, .T. ) ;
#2295=FILL_AREA_STYLE ('',( #4599 ) ) ;
#2303=DIRECTION ( 'NONE',  ( -0.7071067811865469066, 0.000000000000000000, -0.7071067811865482389 ) ) ;
#2310=DIRECTION ( 'NONE',  ( 1.000000000000000000, 0.000000000000000000, 0.000000000000000000 ) ) ;
#2317=ORIENTED_EDGE ( 'NONE', *, *, #2412, .T. ) ;
#2318=CIRCLE ( 'NONE', #793, 22.99999999999998934 ) ;
#2324=AXIS2_PLACEMENT_3D ( 'NONE', #3007, #2949, #3275 ) ;
#2326=CARTESIAN_POINT ( 'NONE',  ( 0.000000000000000000, 0.000000000000000000, -12.00000000000000000 ) ) ;
#2328=CIRCLE ( 'NONE', #639, 23.00000000000000711 ) ;
#2330=ORIENTED_EDGE ( 'NONE', *, *, #2216, .T. ) ;
#2333=VECTOR ( 'NONE', #4016, 1000.000000000000000 ) ;
#2342=VECTOR ( 'NONE', #3419, 1000.000000000000000 ) ;
#2345=VERTEX_POINT ( 'NONE', #4532 ) ;
#2346=CIRCLE ( 'NONE', #983, 25.00000000000000000 ) ;
#2354=VECTOR ( 'NONE', #3273, 1000.000000000000000 ) ;
#2360=ORIENTED_EDGE ( 'NONE', *, *, #4767, .F. ) ;
#2385=EDGE_CURVE ( 'NONE', #4859, #2525, #1862, .T. ) ;
#2398=LINE ( 'NONE', #2051, #4399 ) ;
#2400=EDGE_CURVE ( 'NONE', #1400, #2525, #4087, .T. ) ;
#2403=CARTESIAN_POINT ( 'NONE',  ( -8.500000000000003553, 21.37171027316251681, 12.00000000000000000 ) ) ;
#2407=ORIENTED_EDGE ( 'NONE', *, *, #3872, .F. ) ;
#2412=EDGE_CURVE ( 'NONE', #4052, #1430, #3024, .T. ) ;
#2413=LINE ( 'NONE', #3431, #3224 ) ;
#2425=ORIENTED_EDGE ( 'NONE', *, *, #272, .T. ) ;
#2432=AXIS2_PLACEMENT_3D ( 'NONE', #4240, #454, #1589 ) ;
#2446=DIRECTION ( 'NONE',  ( -0.000000000000000000, 0.000000000000000000, 1.000000000000000000 ) ) ;
#2452=DIRECTION ( 'NONE',  ( 1.106769389831504682E-16, -1.000000000000000000, 0.000000000000000000 ) ) ;
#2453=ORIENTED_EDGE ( 'NONE', *, *, #1385, .F. ) ;
#2455=CARTESIAN_POINT ( 'NONE',  ( 19.30673457630776468, -12.50000000000007105, -4.000000000000000000 ) ) ;
#2463=CARTESIAN_POINT ( 'NONE',  ( 4.196500603111122875E-14, 12.50000000000000178, -12.00000000000000000 ) ) ;
#2471=CARTESIAN_POINT ( 'NONE',  ( 0.000000000000000000, 0.000000000000000000, 12.00000000000000000 ) ) ;
#2484=ORIENTED_EDGE ( 'NONE', *, *, #53, .F. ) ;
#2488=DIRECTION ( 'NONE',  ( -0.000000000000000000, 0.000000000000000000, 1.000000000000000000 ) ) ;
#2490=AXIS2_PLACEMENT_3D ( 'NONE', #453, #3471, #86 ) ;
#2508=ORIENTED_EDGE ( 'NONE', *, *, #4204, .T. ) ;
#2513=CYLINDRICAL_SURFACE ( 'NONE', #4816, 22.99999999999998934 ) ;
#2519=EDGE_LOOP ( 'NONE', ( #3526, #283, #3854 ) ) ;
#2522=CARTESIAN_POINT ( 'NONE',  ( -8.500000000000001776, -9.407539813567788568E-16, 12.00000000000000000 ) ) ;
#2523=AXIS2_PLACEMENT_3D ( 'NONE', #301, #1123, #1074 ) ;
#2525=VERTEX_POINT ( 'NONE', #3867 ) ;
#2543=LINE ( 'NONE', #1409, #4586 ) ;
#2546=PLANE ( 'NONE',  #3360 ) ;
#2549=CARTESIAN_POINT ( 'NONE',  ( 19.30673457630776468, -12.50000000000007105, -12.00000000000000000 ) ) ;
#2551=PRODUCT_DEFINITION_FORMATION_WITH_SPECIFIED_SOURCE ( 'ANY', '', #1668, .NOT_KNOWN. ) ;
#2552=DIRECTION ( 'NONE',  ( 1.000000000000000000, 0.000000000000000000, 0.000000000000000000 ) ) ;
#2564=CARTESIAN_POINT ( 'NONE',  ( 0.000000000000000000, 0.000000000000000000, 4.000000000000000000 ) ) ;
#2567=CARTESIAN_POINT ( 'NONE',  ( 12.50000000000000000, -1.383461737289380927E-15, 12.00000000000000000 ) ) ;
#2576=AXIS2_PLACEMENT_3D ( 'NONE', #1131, #677, #1450 ) ;
#2577=AXIS2_PLACEMENT_3D ( 'NONE', #2868, #3170, #2038 ) ;
#2579=DIRECTION ( 'NONE',  ( 0.000000000000000000, 0.000000000000000000, -1.000000000000000000 ) ) ;
#2584=ADVANCED_FACE ( 'NONE', ( #471 ), #4688, .T. ) ;
#2587=LINE ( 'NONE', #1100, #647 ) ;
#2590=DIRECTION ( 'NONE',  ( -0.000000000000000000, -0.000000000000000000, -1.000000000000000000 ) ) ;
#2603=AXIS2_PLACEMENT_3D ( 'NONE', #4880, #4195, #3819 ) ;
#2616=DIRECTION ( 'NONE',  ( -0.000000000000000000, -0.000000000000000000, -1.000000000000000000 ) ) ;
#2620=EDGE_CURVE ( 'NONE', #3659, #3812, #2045, .T. ) ;
#2621=CARTESIAN_POINT ( 'NONE',  ( 8.500000000000003553, 21.37171027316251681, 4.000000000000000000 ) ) ;
#2632=CARTESIAN_POINT ( 'NONE',  ( -8.500000000000003553, 21.37171027316251681, 12.00000000000000000 ) ) ;
#2634=DIRECTION ( 'NONE',  ( 1.000000000000000000, 1.106769389831504189E-16, -0.000000000000000000 ) ) ;
#2635=ORIENTED_EDGE ( 'NONE', *, *, #2740, .T. ) ;
#2636=CARTESIAN_POINT ( 'NONE',  ( -12.49999999999999822, -19.30673457630782863, 12.00000000000000000 ) ) ;
#2644=ADVANCED_FACE ( 'NONE', ( #1748 ), #982, .F. ) ;
#2649=VECTOR ( 'NONE', #1325, 1000.000000000000000 ) ;
#2653=UNCERTAINTY_MEASURE_WITH_UNIT (LENGTH_MEASURE( 1.000000000000000082E-05 ), #1392, 'distance_accuracy_value', 'NONE');
#2661=CIRCLE ( 'NONE', #2577, 23.00000000000000711 ) ;
#2674=CARTESIAN_POINT ( 'NONE',  ( -8.500000000000000000, -21.37171027316251681, 12.00000000000000000 ) ) ;
#2677=DIRECTION ( 'NONE',  ( 0.000000000000000000, 0.000000000000000000, -1.000000000000000000 ) ) ;
#2685=ADVANCED_FACE ( 'NONE', ( #917 ), #4787, .T. ) ;
#2698=EDGE_LOOP ( 'NONE', ( #697, #1753, #246, #4017 ) ) ;
#2700=DIRECTION ( 'NONE',  ( 0.000000000000000000, 0.000000000000000000, 1.000000000000000000 ) ) ;
#2722=SHAPE_REPRESENTATION_RELATIONSHIP ( 'NONE' , 'NONE' ,  #1644, #38 ) ;
#2724=PLANE ( 'NONE',  #2432 ) ;
#2726=CIRCLE ( 'NONE', #1205, 22.99999999999998934 ) ;
#2734=PRODUCT_DEFINITION_CONTEXT ( 'detailed design', #1723, 'design' ) ;
#2739=DIRECTION ( 'NONE',  ( -0.000000000000000000, -0.000000000000000000, -1.000000000000000000 ) ) ;
#2740=EDGE_CURVE ( 'NONE', #1594, #3321, #3585, .T. ) ;
#2745=CARTESIAN_POINT ( 'NONE',  ( 0.000000000000000000, 0.000000000000000000, -4.000000000000000000 ) ) ;
#2746=DIRECTION ( 'NONE',  ( 0.000000000000000000, 0.000000000000000000, -1.000000000000000000 ) ) ;
#2747=AXIS2_PLACEMENT_3D ( 'NONE', #3345, #2677, #4872 ) ;
#2748=AXIS2_PLACEMENT_3D ( 'NONE', #4689, #3586, #886 ) ;
#2750=ADVANCED_FACE ( 'NONE', ( #4713 ), #4033, .F. ) ;
#2753=AXIS2_PLACEMENT_3D ( 'NONE', #4272, #1076, #4521 ) ;
#2754=ORIENTED_EDGE ( 'NONE', *, *, #2898, .F. ) ;
#2757=CARTESIAN_POINT ( 'NONE',  ( 23.00000000000000711, 2.816687638038913141E-15, 4.000000000000000000 ) ) ;
#2763=DIRECTION ( 'NONE',  ( -1.000000000000000000, 3.357200482488896896E-15, 0.000000000000000000 ) ) ;
#2764=CARTESIAN_POINT ( 'NONE',  ( 0.000000000000000000, 0.000000000000000000, 4.000000000000000000 ) ) ;
#2765=VERTEX_POINT ( 'NONE', #2872 ) ;
#2773=DIRECTION ( 'NONE',  ( -1.000000000000000000, 0.000000000000000000, 0.000000000000000000 ) ) ;
#2780=CARTESIAN_POINT ( 'NONE',  ( 0.000000000000000000, 0.000000000000000000, 12.00000000000000000 ) ) ;
#2793=EDGE_LOOP ( 'NONE', ( #1956, #1348, #3817, #859 ) ) ;
#2795=FACE_OUTER_BOUND ( 'NONE', #2698, .T. ) ;
#2812=CIRCLE ( 'NONE', #1922, 23.00000000000000711 ) ;
#2815=DIRECTION ( 'NONE',  ( 1.000000000000000000, 0.000000000000000000, 0.000000000000000000 ) ) ;
#2816=EDGE_CURVE ( 'NONE', #1313, #4859, #1827, .T. ) ;
#2826=ORIENTED_EDGE ( 'NONE', *, *, #2740, .F. ) ;
#2833=DIRECTION ( 'NONE',  ( -0.000000000000000000, -0.000000000000000000, 1.000000000000000000 ) ) ;
#2840=DIRECTION ( 'NONE',  ( 0.000000000000000000, 0.000000000000000000, 1.000000000000000000 ) ) ;
#2842=ORIENTED_EDGE ( 'NONE', *, *, #2276, .F. ) ;
#2843=CONICAL_SURFACE ( 'NONE', #2192, 25.00000000000000000, 0.7853981633974500554 ) ;
#2845=EDGE_CURVE ( 'NONE', #3988, #3154, #4451, .T. ) ;
#2859=FACE_OUTER_BOUND ( 'NONE', #3243, .T. ) ;
#2861=ORIENTED_EDGE ( 'NONE', *, *, #1577, .F. ) ;
#2866=DIRECTION ( 'NONE',  ( -0.000000000000000000, -0.000000000000000000, -1.000000000000000000 ) ) ;
#2868=CARTESIAN_POINT ( 'NONE',  ( 0.000000000000000000, 0.000000000000000000, 4.000000000000000000 ) ) ;
#2872=CARTESIAN_POINT ( 'NONE',  ( -21.37171027316247063, 8.500000000000072831, -12.00000000000000000 ) ) ;
#2876=ORIENTED_EDGE ( 'NONE', *, *, #907, .F. ) ;
#2878=LINE ( 'NONE', #3252, #4742 ) ;
#2886=DIRECTION ( 'NONE',  ( -0.000000000000000000, -0.000000000000000000, -1.000000000000000000 ) ) ;
#2888=CARTESIAN_POINT ( 'NONE',  ( -3.041771206386918902E-14, -8.500000000000001776, -12.00000000000000000 ) ) ;
#2891=LINE ( 'NONE', #3286, #652 ) ;
#2892=ORIENTED_EDGE ( 'NONE', *, *, #4604, .T. ) ;
#2894=ORIENTED_EDGE ( 'NONE', *, *, #2620, .F. ) ;
#2898=EDGE_CURVE ( 'NONE', #4346, #3611, #1134, .T. ) ;
#2909=AXIS2_PLACEMENT_3D ( 'NONE', #1403, #2938, #4503 ) ;
#2915=CLOSED_SHELL ( 'NONE', ( #2112, #4054, #1571, #421, #4696, #4380, #18, #1019, #914, #1596, #3329, #954, #4447, #1338, #4145, #4756, #2685, #2991, #2644, #3026, #4697, #2197, #3781, #1871, #3444, #1726, #2584, #2111, #2750, #3142, #352, #4875 ) ) ;
#2916=CIRCLE ( 'NONE', #745, 23.00000000000000711 ) ;
#2918=DIRECTION ( 'NONE',  ( -3.357200482488897685E-15, -1.000000000000000000, 0.000000000000000000 ) ) ;
#2919=VERTEX_POINT ( 'NONE', #2188 ) ;
#2923=LINE ( 'NONE', #3971, #4328 ) ;
#2927=CARTESIAN_POINT ( 'NONE',  ( 21.37171027316246708, -8.500000000000078160, -12.00000000000000000 ) ) ;
#2932=DIRECTION ( 'NONE',  ( -1.000000000000000000, 3.357200482488897290E-15, 0.000000000000000000 ) ) ;
#2938=DIRECTION ( 'NONE',  ( 0.000000000000000000, 0.000000000000000000, 1.000000000000000000 ) ) ;
#2945=VERTEX_POINT ( 'NONE', #2283 ) ;
#2949=DIRECTION ( 'NONE',  ( 0.000000000000000000, 0.000000000000000000, -1.000000000000000000 ) ) ;
#2959=VECTOR ( 'NONE', #1623, 1000.000000000000000 ) ;
#2960=DIRECTION ( 'NONE',  ( 3.578554360455198522E-15, 1.000000000000000000, 0.000000000000000000 ) ) ;
#2968=DIRECTION ( 'NONE',  ( 0.000000000000000000, 0.000000000000000000, -1.000000000000000000 ) ) ;
#2972=CARTESIAN_POINT ( 'NONE',  ( 4.196500603111122875E-14, 12.50000000000000178, -4.000000000000000000 ) ) ;
#2973=CIRCLE ( 'NONE', #4476, 22.99999999999998934 ) ;
#2975=LINE ( 'NONE', #4501, #578 ) ;
#2976=CARTESIAN_POINT ( 'NONE',  ( 0.000000000000000000, 0.000000000000000000, -12.00000000000000000 ) ) ;
#2983=EDGE_CURVE ( 'NONE', #1202, #754, #4631, .T. ) ;
#2988=AXIS2_PLACEMENT_3D ( 'NONE', #845, #1250, #4622 ) ;
#2991=ADVANCED_FACE ( 'NONE', ( #3860 ), #403, .T. ) ;
#2997=EDGE_CURVE ( 'NONE', #4073, #3915, #4256, .T. ) ;
#3007=CARTESIAN_POINT ( 'NONE',  ( 0.000000000000000000, 0.000000000000000000, -4.000000000000000000 ) ) ;
#3011=FACE_OUTER_BOUND ( 'NONE', #2154, .T. ) ;
#3016=LINE ( 'NONE', #2632, #743 ) ;
#3019=EDGE_CURVE ( 'NONE', #754, #1649, #2413, .T. ) ;
#3021=ORIENTED_EDGE ( 'NONE', *, *, #1883, .F. ) ;
#3024=LINE ( 'NONE', #1138, #4746 ) ;
#3026=ADVANCED_FACE ( 'NONE', ( #4610 ), #1523, .T. ) ;
#3029=CARTESIAN_POINT ( 'NONE',  ( -12.50000000000000000, -1.383461737289380927E-15, 12.00000000000000000 ) ) ;
#3033=FACE_OUTER_BOUND ( 'NONE', #4283, .T. ) ;
#3040=AXIS2_PLACEMENT_3D ( 'NONE', #1301, #123, #1344 ) ;
#3053=FACE_OUTER_BOUND ( 'NONE', #4928, .T. ) ;
#3057=VECTOR ( 'NONE', #384, 1000.000000000000000 ) ;
#3064=ORIENTED_EDGE ( 'NONE', *, *, #3907, .F. ) ;
#3074=CARTESIAN_POINT ( 'NONE',  ( 0.000000000000000000, 0.000000000000000000, 2.000000000000001776 ) ) ;
#3076=FACE_OUTER_BOUND ( 'NONE', #2519, .T. ) ;
#3082=( NAMED_UNIT ( * ) SI_UNIT ( $, .STERADIAN. ) SOLID_ANGLE_UNIT ( ) );
#3083=PLANE ( 'NONE',  #2490 ) ;
#3097=PRODUCT_DEFINITION_SHAPE ( 'NONE', 'NONE',  #4361 ) ;
#3100=CARTESIAN_POINT ( 'NONE',  ( 25.00000000000000000, 0.000000000000000000, -1.999999999999994893 ) ) ;
#3107=ORIENTED_EDGE ( 'NONE', *, *, #802, .T. ) ;
#3108=DIRECTION ( 'NONE',  ( 0.000000000000000000, 0.000000000000000000, -1.000000000000000000 ) ) ;
#3110=EDGE_CURVE ( 'NONE', #2345, #4346, #490, .T. ) ;
#3111=ORIENTED_EDGE ( 'NONE', *, *, #1095, .F. ) ;
#3127=FILL_AREA_STYLE_COLOUR ( '', #4717 ) ;
#3129=CYLINDRICAL_SURFACE ( 'NONE', #906, 22.99999999999998934 ) ;
#3141=ORIENTED_EDGE ( 'NONE', *, *, #11, .T. ) ;
#3142=ADVANCED_FACE ( 'NONE', ( #3979 ), #2513, .T. ) ;
#3144=VECTOR ( 'NONE', #4771, 1000.000000000000000 ) ;
#3154=VERTEX_POINT ( 'NONE', #4418 ) ;
#3167=CIRCLE ( 'NONE', #2274, 25.00000000000000000 ) ;
#3168=DIRECTION ( 'NONE',  ( 0.000000000000000000, 0.000000000000000000, -1.000000000000000000 ) ) ;
#3170=DIRECTION ( 'NONE',  ( 0.000000000000000000, 0.000000000000000000, 1.000000000000000000 ) ) ;
#3171=DIRECTION ( 'NONE',  ( -0.000000000000000000, -0.000000000000000000, -1.000000000000000000 ) ) ;
#3200=FACE_OUTER_BOUND ( 'NONE', #1702, .T. ) ;
#3201=CARTESIAN_POINT ( 'NONE',  ( 25.00000000000000000, 3.061616997868383043E-15, -1.999999999999994893 ) ) ;
#3220=CIRCLE ( 'NONE', #4567, 22.99999999999998934 ) ;
#3224=VECTOR ( 'NONE', #3171, 1000.000000000000000 ) ;
#3230=LINE ( 'NONE', #590, #2354 ) ;
#3235=CARTESIAN_POINT ( 'NONE',  ( -25.00000000000000000, 0.000000000000000000, 2.000000000000001776 ) ) ;
#3236=CIRCLE ( 'NONE', #4422, 25.00000000000000000 ) ;
#3237=ORIENTED_EDGE ( 'NONE', *, *, #715, .F. ) ;
#3243=EDGE_LOOP ( 'NONE', ( #2292, #1975, #2407, #1391 ) ) ;
#3251=CYLINDRICAL_SURFACE ( 'NONE', #728, 23.00000000000000711 ) ;
#3252=CARTESIAN_POINT ( 'NONE',  ( 21.37171027316252747, 8.499999999999930722, -12.00000000000000000 ) ) ;
#3263=CARTESIAN_POINT ( 'NONE',  ( -25.00000000000000000, 0.000000000000000000, -1.999999999999994893 ) ) ;
#3264=DIRECTION ( 'NONE',  ( 1.000000000000000000, 0.000000000000000000, 0.000000000000000000 ) ) ;
#3272=DIRECTION ( 'NONE',  ( -0.000000000000000000, -0.000000000000000000, 1.000000000000000000 ) ) ;
#3273=DIRECTION ( 'NONE',  ( -1.000000000000000000, 3.357200482488896896E-15, 0.000000000000000000 ) ) ;
#3275=DIRECTION ( 'NONE',  ( -1.000000000000000000, 0.000000000000000000, 0.000000000000000000 ) ) ;
#3279=VECTOR ( 'NONE', #2763, 1000.000000000000000 ) ;
#3280=CARTESIAN_POINT ( 'NONE',  ( 0.000000000000000000, 0.000000000000000000, -12.00000000000000000 ) ) ;
#3282=EDGE_LOOP ( 'NONE', ( #287, #3021, #2453, #1156 ) ) ;
#3284=VECTOR ( 'NONE', #2243, 1000.000000000000000 ) ;
#3286=CARTESIAN_POINT ( 'NONE',  ( 25.00000000000000000, 3.061616997868383043E-15, 4.000000000000000000 ) ) ;
#3303=DIRECTION ( 'NONE',  ( -1.106769389831504313E-16, -1.000000000000000000, 0.000000000000000000 ) ) ;
#3318=EDGE_CURVE ( 'NONE', #4311, #1059, #667, .T. ) ;
#3319=CARTESIAN_POINT ( 'NONE',  ( -22.99999999999998934, 2.939152317953647894E-15, -4.000000000000000000 ) ) ;
#3320=CARTESIAN_POINT ( 'NONE',  ( 12.50000000000000000, -1.383461737289380927E-15, 4.000000000000000000 ) ) ;
#3321=VERTEX_POINT ( 'NONE', #3739 ) ;
#3323=ORIENTED_EDGE ( 'NONE', *, *, #913, .F. ) ;
#3324=ORIENTED_EDGE ( 'NONE', *, *, #1724, .F. ) ;
#3329=ADVANCED_FACE ( 'NONE', ( #293 ), #4899, .T. ) ;
#3331=CARTESIAN_POINT ( 'NONE',  ( 0.000000000000000000, 0.000000000000000000, -4.000000000000000000 ) ) ;
#3338=EDGE_LOOP ( 'NONE', ( #1586, #533, #2508, #3064 ) ) ;
#3344=ORIENTED_EDGE ( 'NONE', *, *, #820, .T. ) ;
#3345=CARTESIAN_POINT ( 'NONE',  ( 0.000000000000000000, 0.000000000000000000, -12.00000000000000000 ) ) ;
#3354=EDGE_CURVE ( 'NONE', #2765, #451, #4013, .T. ) ;
#3355=EDGE_CURVE ( 'NONE', #4459, #4073, #2975, .T. ) ;
#3360=AXIS2_PLACEMENT_3D ( 'NONE', #1070, #993, #614 ) ;
#3362=VECTOR ( 'NONE', #3303, 1000.000000000000000 ) ;
#3363=VERTEX_POINT ( 'NONE', #4200 ) ;
#3380=CONICAL_SURFACE ( 'NONE', #2988, 23.00000000000000711, 0.7853981633974473908 ) ;
#3388=CARTESIAN_POINT ( 'NONE',  ( 21.37171027316252747, 8.499999999999930722, -4.000000000000000000 ) ) ;
#3398=CIRCLE ( 'NONE', #2603, 23.00000000000000711 ) ;
#3403=DIRECTION ( 'NONE',  ( -1.000000000000000000, 0.000000000000000000, 0.000000000000000000 ) ) ;
#3419=DIRECTION ( 'NONE',  ( 1.106769389831504682E-16, -1.000000000000000000, 0.000000000000000000 ) ) ;
#3420=( LENGTH_UNIT ( ) NAMED_UNIT ( * ) SI_UNIT ( .MILLI., .METRE. ) );
#3421=CARTESIAN_POINT ( 'NONE',  ( -8.500000000000001776, -9.407539813567788568E-16, 4.000000000000000000 ) ) ;
#3422=PRESENTATION_STYLE_ASSIGNMENT (( #1868 ) ) ;
#3425=DIRECTION ( 'NONE',  ( 1.000000000000000000, 0.000000000000000000, -0.000000000000000000 ) ) ;
#3431=CARTESIAN_POINT ( 'NONE',  ( -25.00000000000000000, 0.000000000000000000, 4.000000000000000000 ) ) ;
#3432=DIRECTION ( 'NONE',  ( -1.106769389831504189E-16, 1.000000000000000000, 0.000000000000000000 ) ) ;
#3444=ADVANCED_FACE ( 'NONE', ( #2282 ), #4551, .T. ) ;
#3452=ORIENTED_EDGE ( 'NONE', *, *, #2276, .T. ) ;
#3457=CARTESIAN_POINT ( 'NONE',  ( -19.30673457630785350, -12.49999999999993250, -12.00000000000000000 ) ) ;
#3459=AXIS2_PLACEMENT_3D ( 'NONE', #4736, #4708, #1282 ) ;
#3471=DIRECTION ( 'NONE',  ( 0.000000000000000000, 0.000000000000000000, 1.000000000000000000 ) ) ;
#3473=FACE_OUTER_BOUND ( 'NONE', #3973, .T. ) ;
#3477=EDGE_CURVE ( 'NONE', #4758, #553, #3016, .T. ) ;
#3482=ORIENTED_EDGE ( 'NONE', *, *, #2385, .T. ) ;
#3491=DIRECTION ( 'NONE',  ( 0.000000000000000000, 0.000000000000000000, 1.000000000000000000 ) ) ;
#3507=CARTESIAN_POINT ( 'NONE',  ( -19.30673457630776824, 12.50000000000006750, -12.00000000000000000 ) ) ;
#3512=CARTESIAN_POINT ( 'NONE',  ( 0.000000000000000000, 0.000000000000000000, 4.000000000000000000 ) ) ;
#3516=ORIENTED_EDGE ( 'NONE', *, *, #3318, .T. ) ;
#3521=ORIENTED_EDGE ( 'NONE', *, *, #4025, .F. ) ;
#3526=ORIENTED_EDGE ( 'NONE', *, *, #2270, .F. ) ;
#3533=AXIS2_PLACEMENT_3D ( 'NONE', #3542, #3866, #1985 ) ;
#3539=CIRCLE ( 'NONE', #1373, 22.99999999999998934 ) ;
#3542=CARTESIAN_POINT ( 'NONE',  ( 0.000000000000000000, 0.000000000000000000, 4.000000000000000000 ) ) ;
#3544=CARTESIAN_POINT ( 'NONE',  ( 0.000000000000000000, 0.000000000000000000, 12.00000000000000000 ) ) ;
#3546=EDGE_CURVE ( 'NONE', #451, #374, #2039, .T. ) ;
#3547=AXIS2_PLACEMENT_3D ( 'NONE', #1677, #4308, #556 ) ;
#3549=DIRECTION ( 'NONE',  ( -0.000000000000000000, -0.000000000000000000, -1.000000000000000000 ) ) ;
#3556=ORIENTED_EDGE ( 'NONE', *, *, #548, .T. ) ;
#3560=EDGE_CURVE ( 'NONE', #406, #1430, #1780, .T. ) ;
#3565=DIRECTION ( 'NONE',  ( 1.000000000000000000, 0.000000000000000000, 0.000000000000000000 ) ) ;
#3570=FACE_OUTER_BOUND ( 'NONE', #125, .T. ) ;
#3572=EDGE_CURVE ( 'NONE', #553, #4747, #1062, .T. ) ;
#3585=LINE ( 'NONE', #936, #3144 ) ;
#3586=DIRECTION ( 'NONE',  ( 1.000000000000000000, 1.106769389831504682E-16, -0.000000000000000000 ) ) ;
#3604=AXIS2_PLACEMENT_3D ( 'NONE', #445, #2746, #1167 ) ;
#3607=CARTESIAN_POINT ( 'NONE',  ( 8.500000000000001776, -9.407539813567788568E-16, 12.00000000000000000 ) ) ;
#3611=VERTEX_POINT ( 'NONE', #179 ) ;
#3622=LINE ( 'NONE', #4566, #3284 ) ;
#3629=EDGE_CURVE ( 'NONE', #1649, #3812, #2346, .T. ) ;
#3630=ORIENTED_EDGE ( 'NONE', *, *, #802, .F. ) ;
#3638=CARTESIAN_POINT ( 'NONE',  ( -23.00000000000000711, 0.000000000000000000, 4.000000000000000000 ) ) ;
#3639=LINE ( 'NONE', #3320, #4648 ) ;
#3641=DIRECTION ( 'NONE',  ( -0.000000000000000000, -0.000000000000000000, 1.000000000000000000 ) ) ;
#3642=ORIENTED_EDGE ( 'NONE', *, *, #4142, .F. ) ;
#3649=LINE ( 'NONE', #514, #4571 ) ;
#3659=VERTEX_POINT ( 'NONE', #4241 ) ;
#3663=ORIENTED_EDGE ( 'NONE', *, *, #2216, .F. ) ;
#3670=DIRECTION ( 'NONE',  ( 1.000000000000000000, 0.000000000000000000, 0.000000000000000000 ) ) ;
#3692=VERTEX_POINT ( 'NONE', #846 ) ;
#3693=AXIS2_PLACEMENT_3D ( 'NONE', #2174, #1040, #4538 ) ;
#3694=AXIS2_PLACEMENT_3D ( 'NONE', #3544, #2488, #3565 ) ;
#3714=DIRECTION ( 'NONE',  ( -0.000000000000000000, -0.000000000000000000, -1.000000000000000000 ) ) ;
#3718=ORIENTED_EDGE ( 'NONE', *, *, #3572, .F. ) ;
#3725=EDGE_CURVE ( 'NONE', #1262, #374, #1625, .T. ) ;
#3728=CYLINDRICAL_SURFACE ( 'NONE', #4345, 22.99999999999998934 ) ;
#3732=EDGE_LOOP ( 'NONE', ( #4139, #1898, #2263, #3344 ) ) ;
#3738=ORIENTED_EDGE ( 'NONE', *, *, #4025, .T. ) ;
#3739=CARTESIAN_POINT ( 'NONE',  ( 12.50000000000000178, 19.30673457630782863, 4.000000000000000000 ) ) ;
#3771=AXIS2_PLACEMENT_3D ( 'NONE', #2888, #4032, #581 ) ;
#3781=ADVANCED_FACE ( 'NONE', ( #3473 ), #3728, .T. ) ;
#3783=DIRECTION ( 'NONE',  ( -1.106769389831504313E-16, -1.000000000000000000, 0.000000000000000000 ) ) ;
#3793=CARTESIAN_POINT ( 'NONE',  ( 0.000000000000000000, 0.000000000000000000, 4.000000000000000000 ) ) ;
#3812=VERTEX_POINT ( 'NONE', #3201 ) ;
#3813=( NAMED_UNIT ( * ) SI_UNIT ( $, .STERADIAN. ) SOLID_ANGLE_UNIT ( ) );
#3814=DIRECTION ( 'NONE',  ( -0.000000000000000000, -0.000000000000000000, -1.000000000000000000 ) ) ;
#3817=ORIENTED_EDGE ( 'NONE', *, *, #3019, .T. ) ;
#3819=DIRECTION ( 'NONE',  ( 1.000000000000000000, 0.000000000000000000, 0.000000000000000000 ) ) ;
#3821=ORIENTED_EDGE ( 'NONE', *, *, #4860, .F. ) ;
#3830=EDGE_LOOP ( 'NONE', ( #4528, #858, #3237, #192 ) ) ;
#3837=EDGE_CURVE ( 'NONE', #4443, #1262, #3230, .T. ) ;
#3841=ORIENTED_EDGE ( 'NONE', *, *, #3110, .T. ) ;
#3843=DIRECTION ( 'NONE',  ( 1.000000000000000000, 0.000000000000000000, 0.000000000000000000 ) ) ;
#3846=AXIS2_PLACEMENT_3D ( 'NONE', #3793, #3814, #4143 ) ;
#3849=AXIS2_PLACEMENT_3D ( 'NONE', #1530, #444, #2773 ) ;
#3854=ORIENTED_EDGE ( 'NONE', *, *, #535, .T. ) ;
#3860=FACE_OUTER_BOUND ( 'NONE', #1804, .T. ) ;
#3862=ORIENTED_EDGE ( 'NONE', *, *, #3477, .F. ) ;
#3864=EDGE_CURVE ( 'NONE', #3812, #1649, #3236, .T. ) ;
#3866=DIRECTION ( 'NONE',  ( 0.000000000000000000, 0.000000000000000000, 1.000000000000000000 ) ) ;
#3867=CARTESIAN_POINT ( 'NONE',  ( 21.37171027316246708, -8.500000000000078160, -4.000000000000000000 ) ) ;
#3869=ORIENTED_EDGE ( 'NONE', *, *, #1385, .T. ) ;
#3872=EDGE_CURVE ( 'NONE', #4758, #4311, #2916, .T. ) ;
#3885=DIRECTION ( 'NONE',  ( -0.000000000000000000, -0.000000000000000000, -1.000000000000000000 ) ) ;
#3888=CARTESIAN_POINT ( 'NONE',  ( 0.000000000000000000, 0.000000000000000000, -4.000000000000000000 ) ) ;
#3894=DIRECTION ( 'NONE',  ( 0.000000000000000000, 0.000000000000000000, 1.000000000000000000 ) ) ;
#3907=EDGE_CURVE ( 'NONE', #1594, #2345, #1863, .T. ) ;
#3908=ORIENTED_EDGE ( 'NONE', *, *, #2983, .T. ) ;
#3915=VERTEX_POINT ( 'NONE', #1088 ) ;
#3916=AXIS2_PLACEMENT_3D ( 'NONE', #1973, #372, #3425 ) ;
#3934=CIRCLE ( 'NONE', #3533, 23.00000000000000711 ) ;
#3936=EDGE_LOOP ( 'NONE', ( #4011, #2285, #4117, #3141 ) ) ;
#3953=ORIENTED_EDGE ( 'NONE', *, *, #4832, .T. ) ;
#3957=CIRCLE ( 'NONE', #1870, 25.00000000000000000 ) ;
#3967=EDGE_CURVE ( 'NONE', #803, #3915, #2543, .T. ) ;
#3971=CARTESIAN_POINT ( 'NONE',  ( -12.50000000000000000, -1.383461737289380927E-15, 4.000000000000000000 ) ) ;
#3972=EDGE_CURVE ( 'NONE', #374, #2945, #1429, .T. ) ;
#3973=EDGE_LOOP ( 'NONE', ( #785, #1998, #4951, #3482 ) ) ;
#3975=CARTESIAN_POINT ( 'NONE',  ( 8.500000000000001776, -9.407539813567788568E-16, 12.00000000000000000 ) ) ;
#3979=FACE_OUTER_BOUND ( 'NONE', #4423, .T. ) ;
#3988=VERTEX_POINT ( 'NONE', #2621 ) ;
#4005=FACE_OUTER_BOUND ( 'NONE', #4906, .T. ) ;
#4006=DIRECTION ( 'NONE',  ( 1.106769389831504189E-16, 1.000000000000000000, 0.000000000000000000 ) ) ;
#4008=AXIS2_PLACEMENT_3D ( 'NONE', #4431, #2446, #3264 ) ;
#4011=ORIENTED_EDGE ( 'NONE', *, *, #3560, .T. ) ;
#4013=CIRCLE ( 'NONE', #2747, 22.99999999999998934 ) ;
#4016=DIRECTION ( 'NONE',  ( 1.106769389831504313E-16, -1.000000000000000000, 0.000000000000000000 ) ) ;
#4017=ORIENTED_EDGE ( 'NONE', *, *, #3019, .F. ) ;
#4022=LINE ( 'NONE', #3975, #3362 ) ;
#4025=EDGE_CURVE ( 'NONE', #374, #2945, #585, .T. ) ;
#4032=DIRECTION ( 'NONE',  ( -3.578554360455197734E-15, -1.000000000000000000, 0.000000000000000000 ) ) ;
#4033=PLANE ( 'NONE',  #505 ) ;
#4035=ORIENTED_EDGE ( 'NONE', *, *, #2983, .F. ) ;
#4052=VERTEX_POINT ( 'NONE', #2674 ) ;
#4053=CARTESIAN_POINT ( 'NONE',  ( -4.473192950568998942E-14, -12.50000000000000178, -12.00000000000000000 ) ) ;
#4054=ADVANCED_FACE ( 'NONE', ( #4950 ), #2843, .T. ) ;
#4072=PLANE ( 'NONE',  #4918 ) ;
#4073=VERTEX_POINT ( 'NONE', #1112 ) ;
#4084=DIRECTION ( 'NONE',  ( 1.000000000000000000, 0.000000000000000000, -0.000000000000000000 ) ) ;
#4087=LINE ( 'NONE', #683, #3057 ) ;
#4089=ORIENTED_EDGE ( 'NONE', *, *, #3967, .F. ) ;
#4097=DIRECTION ( 'NONE',  ( -1.000000000000000000, 0.000000000000000000, 0.000000000000000000 ) ) ;
#4098=FACE_OUTER_BOUND ( 'NONE', #2793, .T. ) ;
#4101=ORIENTED_EDGE ( 'NONE', *, *, #2261, .T. ) ;
#4107=FACE_OUTER_BOUND ( 'NONE', #3732, .T. ) ;
#4113=DIRECTION ( 'NONE',  ( -1.000000000000000000, 0.000000000000000000, 0.000000000000000000 ) ) ;
#4114=DIRECTION ( 'NONE',  ( -0.000000000000000000, -0.000000000000000000, 1.000000000000000000 ) ) ;
#4117=ORIENTED_EDGE ( 'NONE', *, *, #450, .F. ) ;
#4120=CARTESIAN_POINT ( 'NONE',  ( 0.000000000000000000, 0.000000000000000000, 4.000000000000000000 ) ) ;
#4134=CARTESIAN_POINT ( 'NONE',  ( -21.37171027316253102, -8.499999999999925393, -4.000000000000000000 ) ) ;
#4137=ORIENTED_EDGE ( 'NONE', *, *, #3972, .F. ) ;
#4139=ORIENTED_EDGE ( 'NONE', *, *, #3967, .T. ) ;
#4142=EDGE_CURVE ( 'NONE', #2765, #1262, #4342, .T. ) ;
#4143=DIRECTION ( 'NONE',  ( -1.000000000000000000, 0.000000000000000000, 0.000000000000000000 ) ) ;
#4144=ORIENTED_EDGE ( 'NONE', *, *, #379, .T. ) ;
#4145=ADVANCED_FACE ( 'NONE', ( #2068 ), #4667, .F. ) ;
#4147=CARTESIAN_POINT ( 'NONE',  ( 0.000000000000000000, 0.000000000000000000, -4.000000000000000000 ) ) ;
#4151=DIRECTION ( 'NONE',  ( -0.000000000000000000, -0.000000000000000000, -1.000000000000000000 ) ) ;
#4156=LINE ( 'NONE', #2636, #836 ) ;
#4161=VECTOR ( 'NONE', #1616, 999.9999999999998863 ) ;
#4165=DIRECTION ( 'NONE',  ( 1.106769389831504313E-16, -1.000000000000000000, 0.000000000000000000 ) ) ;
#4169=PLANE ( 'NONE',  #76 ) ;
#4191=SURFACE_SIDE_STYLE ('',( #1507 ) ) ;
#4192=LINE ( 'NONE', #3421, #1212 ) ;
#4195=DIRECTION ( 'NONE',  ( -0.000000000000000000, 0.000000000000000000, 1.000000000000000000 ) ) ;
#4200=CARTESIAN_POINT ( 'NONE',  ( 19.30673457630784995, 12.49999999999993783, -12.00000000000000000 ) ) ;
#4204=EDGE_CURVE ( 'NONE', #4243, #2345, #4741, .T. ) ;
#4209=ORIENTED_EDGE ( 'NONE', *, *, #1551, .F. ) ;
#4230=STYLED_ITEM ( 'NONE', ( #1587 ), #38 ) ;
#4231=DIRECTION ( 'NONE',  ( -0.000000000000000000, -0.000000000000000000, -1.000000000000000000 ) ) ;
#4240=CARTESIAN_POINT ( 'NONE',  ( 0.000000000000000000, 0.000000000000000000, 12.00000000000000000 ) ) ;
#4241=CARTESIAN_POINT ( 'NONE',  ( 22.99999999999998934, 0.000000000000000000, -4.000000000000000000 ) ) ;
#4243=VERTEX_POINT ( 'NONE', #650 ) ;
#4251=ORIENTED_EDGE ( 'NONE', *, *, #2400, .F. ) ;
#4256=LINE ( 'NONE', #3457, #1444 ) ;
#4263=EDGE_CURVE ( 'NONE', #3692, #3812, #2891, .T. ) ;
#4272=CARTESIAN_POINT ( 'NONE',  ( 0.000000000000000000, 0.000000000000000000, -4.000000000000000000 ) ) ;
#4283=EDGE_LOOP ( 'NONE', ( #4137, #3738 ) ) ;
#4285=DIRECTION ( 'NONE',  ( 1.000000000000000000, 0.000000000000000000, 0.000000000000000000 ) ) ;
#4291=ORIENTED_EDGE ( 'NONE', *, *, #4767, .T. ) ;
#4293=DIRECTION ( 'NONE',  ( 1.000000000000000000, 0.000000000000000000, 0.000000000000000000 ) ) ;
#4294=DIRECTION ( 'NONE',  ( -0.000000000000000000, 0.000000000000000000, 1.000000000000000000 ) ) ;
#4308=DIRECTION ( 'NONE',  ( -0.000000000000000000, 0.000000000000000000, 1.000000000000000000 ) ) ;
#4311=VERTEX_POINT ( 'NONE', #678 ) ;
#4328=VECTOR ( 'NONE', #2452, 1000.000000000000000 ) ;
#4342=LINE ( 'NONE', #1711, #1533 ) ;
#4345=AXIS2_PLACEMENT_3D ( 'NONE', #302, #2833, #2099 ) ;
#4346=VERTEX_POINT ( 'NONE', #4889 ) ;
#4353=CARTESIAN_POINT ( 'NONE',  ( -25.00000000000000000, 3.061616997868383043E-15, -1.999999999999994893 ) ) ;
#4355=AXIS2_PLACEMENT_3D ( 'NONE', #4147, #1548, #767 ) ;
#4356=EDGE_CURVE ( 'NONE', #3611, #3321, #1057, .T. ) ;
#4361=PRODUCT_DEFINITION ( 'UNKNOWN', '', #2551, #2734 ) ;
#4363=CARTESIAN_POINT ( 'NONE',  ( 0.000000000000000000, 0.000000000000000000, -4.000000000000000000 ) ) ;
#4366=ORIENTED_EDGE ( 'NONE', *, *, #2400, .T. ) ;
#4369=CARTESIAN_POINT ( 'NONE',  ( 0.000000000000000000, 0.000000000000000000, 12.00000000000000000 ) ) ;
#4380=ADVANCED_FACE ( 'NONE', ( #725 ), #1856, .F. ) ;
#4399=VECTOR ( 'NONE', #3549, 1000.000000000000000 ) ;
#4400=ORIENTED_EDGE ( 'NONE', *, *, #2845, .F. ) ;
#4415=DIRECTION ( 'NONE',  ( -1.000000000000000000, 3.578554360455198522E-15, 0.000000000000000000 ) ) ;
#4418=CARTESIAN_POINT ( 'NONE',  ( 8.500000000000000000, -21.37171027316251681, 4.000000000000000000 ) ) ;
#4422=AXIS2_PLACEMENT_3D ( 'NONE', #944, #3641, #1359 ) ;
#4423=EDGE_LOOP ( 'NONE', ( #760, #3663, #456, #1751 ) ) ;
#4425=CARTESIAN_POINT ( 'NONE',  ( 0.000000000000000000, 0.000000000000000000, -4.000000000000000000 ) ) ;
#4431=CARTESIAN_POINT ( 'NONE',  ( 0.000000000000000000, 0.000000000000000000, 12.00000000000000000 ) ) ;
#4432=ORIENTED_EDGE ( 'NONE', *, *, #1976, .F. ) ;
#4435=DIRECTION ( 'NONE',  ( -1.106769389831504682E-16, -1.000000000000000000, 0.000000000000000000 ) ) ;
#4436=CARTESIAN_POINT ( 'NONE',  ( 0.000000000000000000, 0.000000000000000000, -4.000000000000000000 ) ) ;
#4438=ORIENTED_EDGE ( 'NONE', *, *, #2898, .T. ) ;
#4443=VERTEX_POINT ( 'NONE', #3388 ) ;
#4447=ADVANCED_FACE ( 'NONE', ( #1104 ), #1881, .T. ) ;
#4451=LINE ( 'NONE', #4863, #4810 ) ;
#4455=FACE_OUTER_BOUND ( 'NONE', #4544, .T. ) ;
#4459=VERTEX_POINT ( 'NONE', #2549 ) ;
#4465=DIRECTION ( 'NONE',  ( 0.000000000000000000, 0.000000000000000000, -1.000000000000000000 ) ) ;
#4476=AXIS2_PLACEMENT_3D ( 'NONE', #2223, #1465, #1818 ) ;
#4500=DIRECTION ( 'NONE',  ( -1.000000000000000000, 3.578554360455198522E-15, 0.000000000000000000 ) ) ;
#4501=CARTESIAN_POINT ( 'NONE',  ( -4.473192950568998942E-14, -12.50000000000000178, -12.00000000000000000 ) ) ;
#4503=DIRECTION ( 'NONE',  ( 1.000000000000000000, 0.000000000000000000, 0.000000000000000000 ) ) ;
#4513=ORIENTED_EDGE ( 'NONE', *, *, #548, .F. ) ;
#4521=DIRECTION ( 'NONE',  ( -1.000000000000000000, 0.000000000000000000, 0.000000000000000000 ) ) ;
#4525=DIRECTION ( 'NONE',  ( -1.000000000000000000, 3.578554360455198522E-15, 0.000000000000000000 ) ) ;
#4528=ORIENTED_EDGE ( 'NONE', *, *, #2845, .T. ) ;
#4529=DIRECTION ( 'NONE',  ( 1.000000000000000000, 0.000000000000000000, 0.000000000000000000 ) ) ;
#4532=CARTESIAN_POINT ( 'NONE',  ( 12.49999999999999822, -19.30673457630782863, 12.00000000000000000 ) ) ;
#4538=DIRECTION ( 'NONE',  ( 1.000000000000000000, 0.000000000000000000, 0.000000000000000000 ) ) ;
#4544=EDGE_LOOP ( 'NONE', ( #4438, #4686, #3452 ) ) ;
#4546=DIRECTION ( 'NONE',  ( 1.106769389831504682E-16, 1.000000000000000000, 0.000000000000000000 ) ) ;
#4551=CYLINDRICAL_SURFACE ( 'NONE', #1537, 22.99999999999998934 ) ;
#4556=CONICAL_SURFACE ( 'NONE', #2247, 23.00000000000000711, 0.7853981633974473908 ) ;
#4560=DIRECTION ( 'NONE',  ( 1.000000000000000000, 0.000000000000000000, 0.000000000000000000 ) ) ;
#4566=CARTESIAN_POINT ( 'NONE',  ( -12.50000000000000178, 19.30673457630782863, 12.00000000000000000 ) ) ;
#4567=AXIS2_PLACEMENT_3D ( 'NONE', #3888, #4231, #861 ) ;
#4571=VECTOR ( 'NONE', #2886, 1000.000000000000000 ) ;
#4575=AXIS2_PLACEMENT_3D ( 'NONE', #753, #2634, #3432 ) ;
#4576=MECHANICAL_DESIGN_GEOMETRIC_PRESENTATION_REPRESENTATION('',(#1538),#823);
#4586=VECTOR ( 'NONE', #4415, 1000.000000000000000 ) ;
#4587=CARTESIAN_POINT ( 'NONE',  ( 0.000000000000000000, 0.000000000000000000, -4.000000000000000000 ) ) ;
#4595=AXIS2_PLACEMENT_3D ( 'NONE', #3280, #2579, #1419 ) ;
#4599=FILL_AREA_STYLE_COLOUR ( '', #1454 ) ;
#4602=UNCERTAINTY_MEASURE_WITH_UNIT (LENGTH_MEASURE( 1.000000000000000082E-05 ), #3420, 'distance_accuracy_value', 'NONE');
#4604=EDGE_CURVE ( 'NONE', #4073, #1313, #1505, .T. ) ;
#4605=ORIENTED_EDGE ( 'NONE', *, *, #2816, .F. ) ;
#4606=EDGE_CURVE ( 'NONE', #212, #2765, #458, .T. ) ;
#4610=FACE_OUTER_BOUND ( 'NONE', #1639, .T. ) ;
#4615=DIRECTION ( 'NONE',  ( -0.000000000000000000, -0.000000000000000000, -1.000000000000000000 ) ) ;
#4622=DIRECTION ( 'NONE',  ( -1.000000000000000000, 0.000000000000000000, 0.000000000000000000 ) ) ;
#4627=ORIENTED_EDGE ( 'NONE', *, *, #2620, .T. ) ;
#4631=LINE ( 'NONE', #1184, #337 ) ;
#4635=MECHANICAL_DESIGN_GEOMETRIC_PRESENTATION_REPRESENTATION('',(#4230),#1821);
#4647=ORIENTED_EDGE ( 'NONE', *, *, #3318, .F. ) ;
#4648=VECTOR ( 'NONE', #4435, 1000.000000000000000 ) ;
#4649=AXIS2_PLACEMENT_3D ( 'NONE', #2745, #4615, #4285 ) ;
#4659=DIRECTION ( 'NONE',  ( -1.000000000000000000, 0.000000000000000000, 0.000000000000000000 ) ) ;
#4667=PLANE ( 'NONE',  #2748 ) ;
#4672=LINE ( 'NONE', #2757, #4161 ) ;
#4676=EDGE_LOOP ( 'NONE', ( #2101, #1563, #3516, #1105 ) ) ;
#4677=CIRCLE ( 'NONE', #2523, 23.00000000000000711 ) ;
#4686=ORIENTED_EDGE ( 'NONE', *, *, #4356, .T. ) ;
#4688=PLANE ( 'NONE',  #3604 ) ;
#4689=CARTESIAN_POINT ( 'NONE',  ( -12.50000000000000000, -1.383461737289380927E-15, 12.00000000000000000 ) ) ;
#4691=EDGE_LOOP ( 'NONE', ( #3630, #2144, #3324, #635, #2861, #1984, #4627, #1679 ) ) ;
#4696=ADVANCED_FACE ( 'NONE', ( #3033 ), #1175, .F. ) ;
#4697=ADVANCED_FACE ( 'NONE', ( #1199 ), #4169, .T. ) ;
#4700=CARTESIAN_POINT ( 'NONE',  ( -8.500000000000003553, 21.37171027316251681, 4.000000000000000000 ) ) ;
#4708=DIRECTION ( 'NONE',  ( -0.000000000000000000, 0.000000000000000000, 1.000000000000000000 ) ) ;
#4713=FACE_OUTER_BOUND ( 'NONE', #3282, .T. ) ;
#4717=COLOUR_RGB ( '', 0.40784314, 0.44705882, 0.49803922) ;
#4725=ORIENTED_EDGE ( 'NONE', *, *, #11, .F. ) ;
#4730=ORIENTED_EDGE ( 'NONE', *, *, #3907, .T. ) ;
#4736=CARTESIAN_POINT ( 'NONE',  ( 0.000000000000000000, 0.000000000000000000, 4.000000000000000000 ) ) ;
#4741=CIRCLE ( 'NONE', #3694, 23.00000000000000711 ) ;
#4742=VECTOR ( 'NONE', #3272, 1000.000000000000000 ) ;
#4744=VECTOR ( 'NONE', #1575, 1000.000000000000000 ) ;
#4746=VECTOR ( 'NONE', #1111, 1000.000000000000000 ) ;
#4747=VERTEX_POINT ( 'NONE', #167 ) ;
#4756=ADVANCED_FACE ( 'NONE', ( #550 ), #2076, .T. ) ;
#4758=VERTEX_POINT ( 'NONE', #2403 ) ;
#4767=EDGE_CURVE ( 'NONE', #1313, #1400, #93, .T. ) ;
#4771=DIRECTION ( 'NONE',  ( -0.000000000000000000, -0.000000000000000000, -1.000000000000000000 ) ) ;
#4787=PLANE ( 'NONE',  #4008 ) ;
#4797=EDGE_CURVE ( 'NONE', #1443, #1262, #2318, .T. ) ;
#4810=VECTOR ( 'NONE', #3783, 1000.000000000000000 ) ;
#4816=AXIS2_PLACEMENT_3D ( 'NONE', #205, #224, #2815 ) ;
#4832=EDGE_CURVE ( 'NONE', #3363, #212, #2726, .T. ) ;
#4835=FACE_OUTER_BOUND ( 'NONE', #933, .T. ) ;
#4845=CARTESIAN_POINT ( 'NONE',  ( 4.196500603111122875E-14, 12.50000000000000178, -12.00000000000000000 ) ) ;
#4858=DIRECTION ( 'NONE',  ( -0.000000000000000000, -0.000000000000000000, -1.000000000000000000 ) ) ;
#4859=VERTEX_POINT ( 'NONE', #2927 ) ;
#4860=EDGE_CURVE ( 'NONE', #2945, #4443, #1834, .T. ) ;
#4863=CARTESIAN_POINT ( 'NONE',  ( 8.500000000000001776, -9.407539813567788568E-16, 4.000000000000000000 ) ) ;
#4872=DIRECTION ( 'NONE',  ( -1.000000000000000000, 0.000000000000000000, 0.000000000000000000 ) ) ;
#4874=LINE ( 'NONE', #1488, #1759 ) ;
#4875=ADVANCED_FACE ( 'NONE', ( #1464 ), #2546, .T. ) ;
#4880=CARTESIAN_POINT ( 'NONE',  ( 0.000000000000000000, 0.000000000000000000, 4.000000000000000000 ) ) ;
#4889=CARTESIAN_POINT ( 'NONE',  ( 12.49999999999999822, -19.30673457630782863, 4.000000000000000000 ) ) ;
#4895=AXIS2_PLACEMENT_3D ( 'NONE', #1556, #3885, #1236 ) ;
#4897=AXIS2_PLACEMENT_3D ( 'NONE', #4053, #2960, #4500 ) ;
#4899=CONICAL_SURFACE ( 'NONE', #3693, 25.00000000000000000, 0.7853981633974500554 ) ;
#4904=( LENGTH_UNIT ( ) NAMED_UNIT ( * ) SI_UNIT ( .MILLI., .METRE. ) );
#4906=EDGE_LOOP ( 'NONE', ( #4366, #1180, #4605, #4291 ) ) ;
#4918=AXIS2_PLACEMENT_3D ( 'NONE', #203, #1398, #2932 ) ;
#4927=ORIENTED_EDGE ( 'NONE', *, *, #4797, .T. ) ;
#4928=EDGE_LOOP ( 'NONE', ( #2149, #2754, #1005, #3111, #1882, #2117, #3908, #542 ) ) ;
#4933=ORIENTED_EDGE ( 'NONE', *, *, #2131, .F. ) ;
#4950=FACE_OUTER_BOUND ( 'NONE', #1736, .T. ) ;
#4951=ORIENTED_EDGE ( 'NONE', *, *, #272, .F. ) ;
#4953=DIRECTION ( 'NONE',  ( 0.000000000000000000, 0.000000000000000000, -1.000000000000000000 ) ) ;
ENDSEC;
END-ISO-10303-21;
